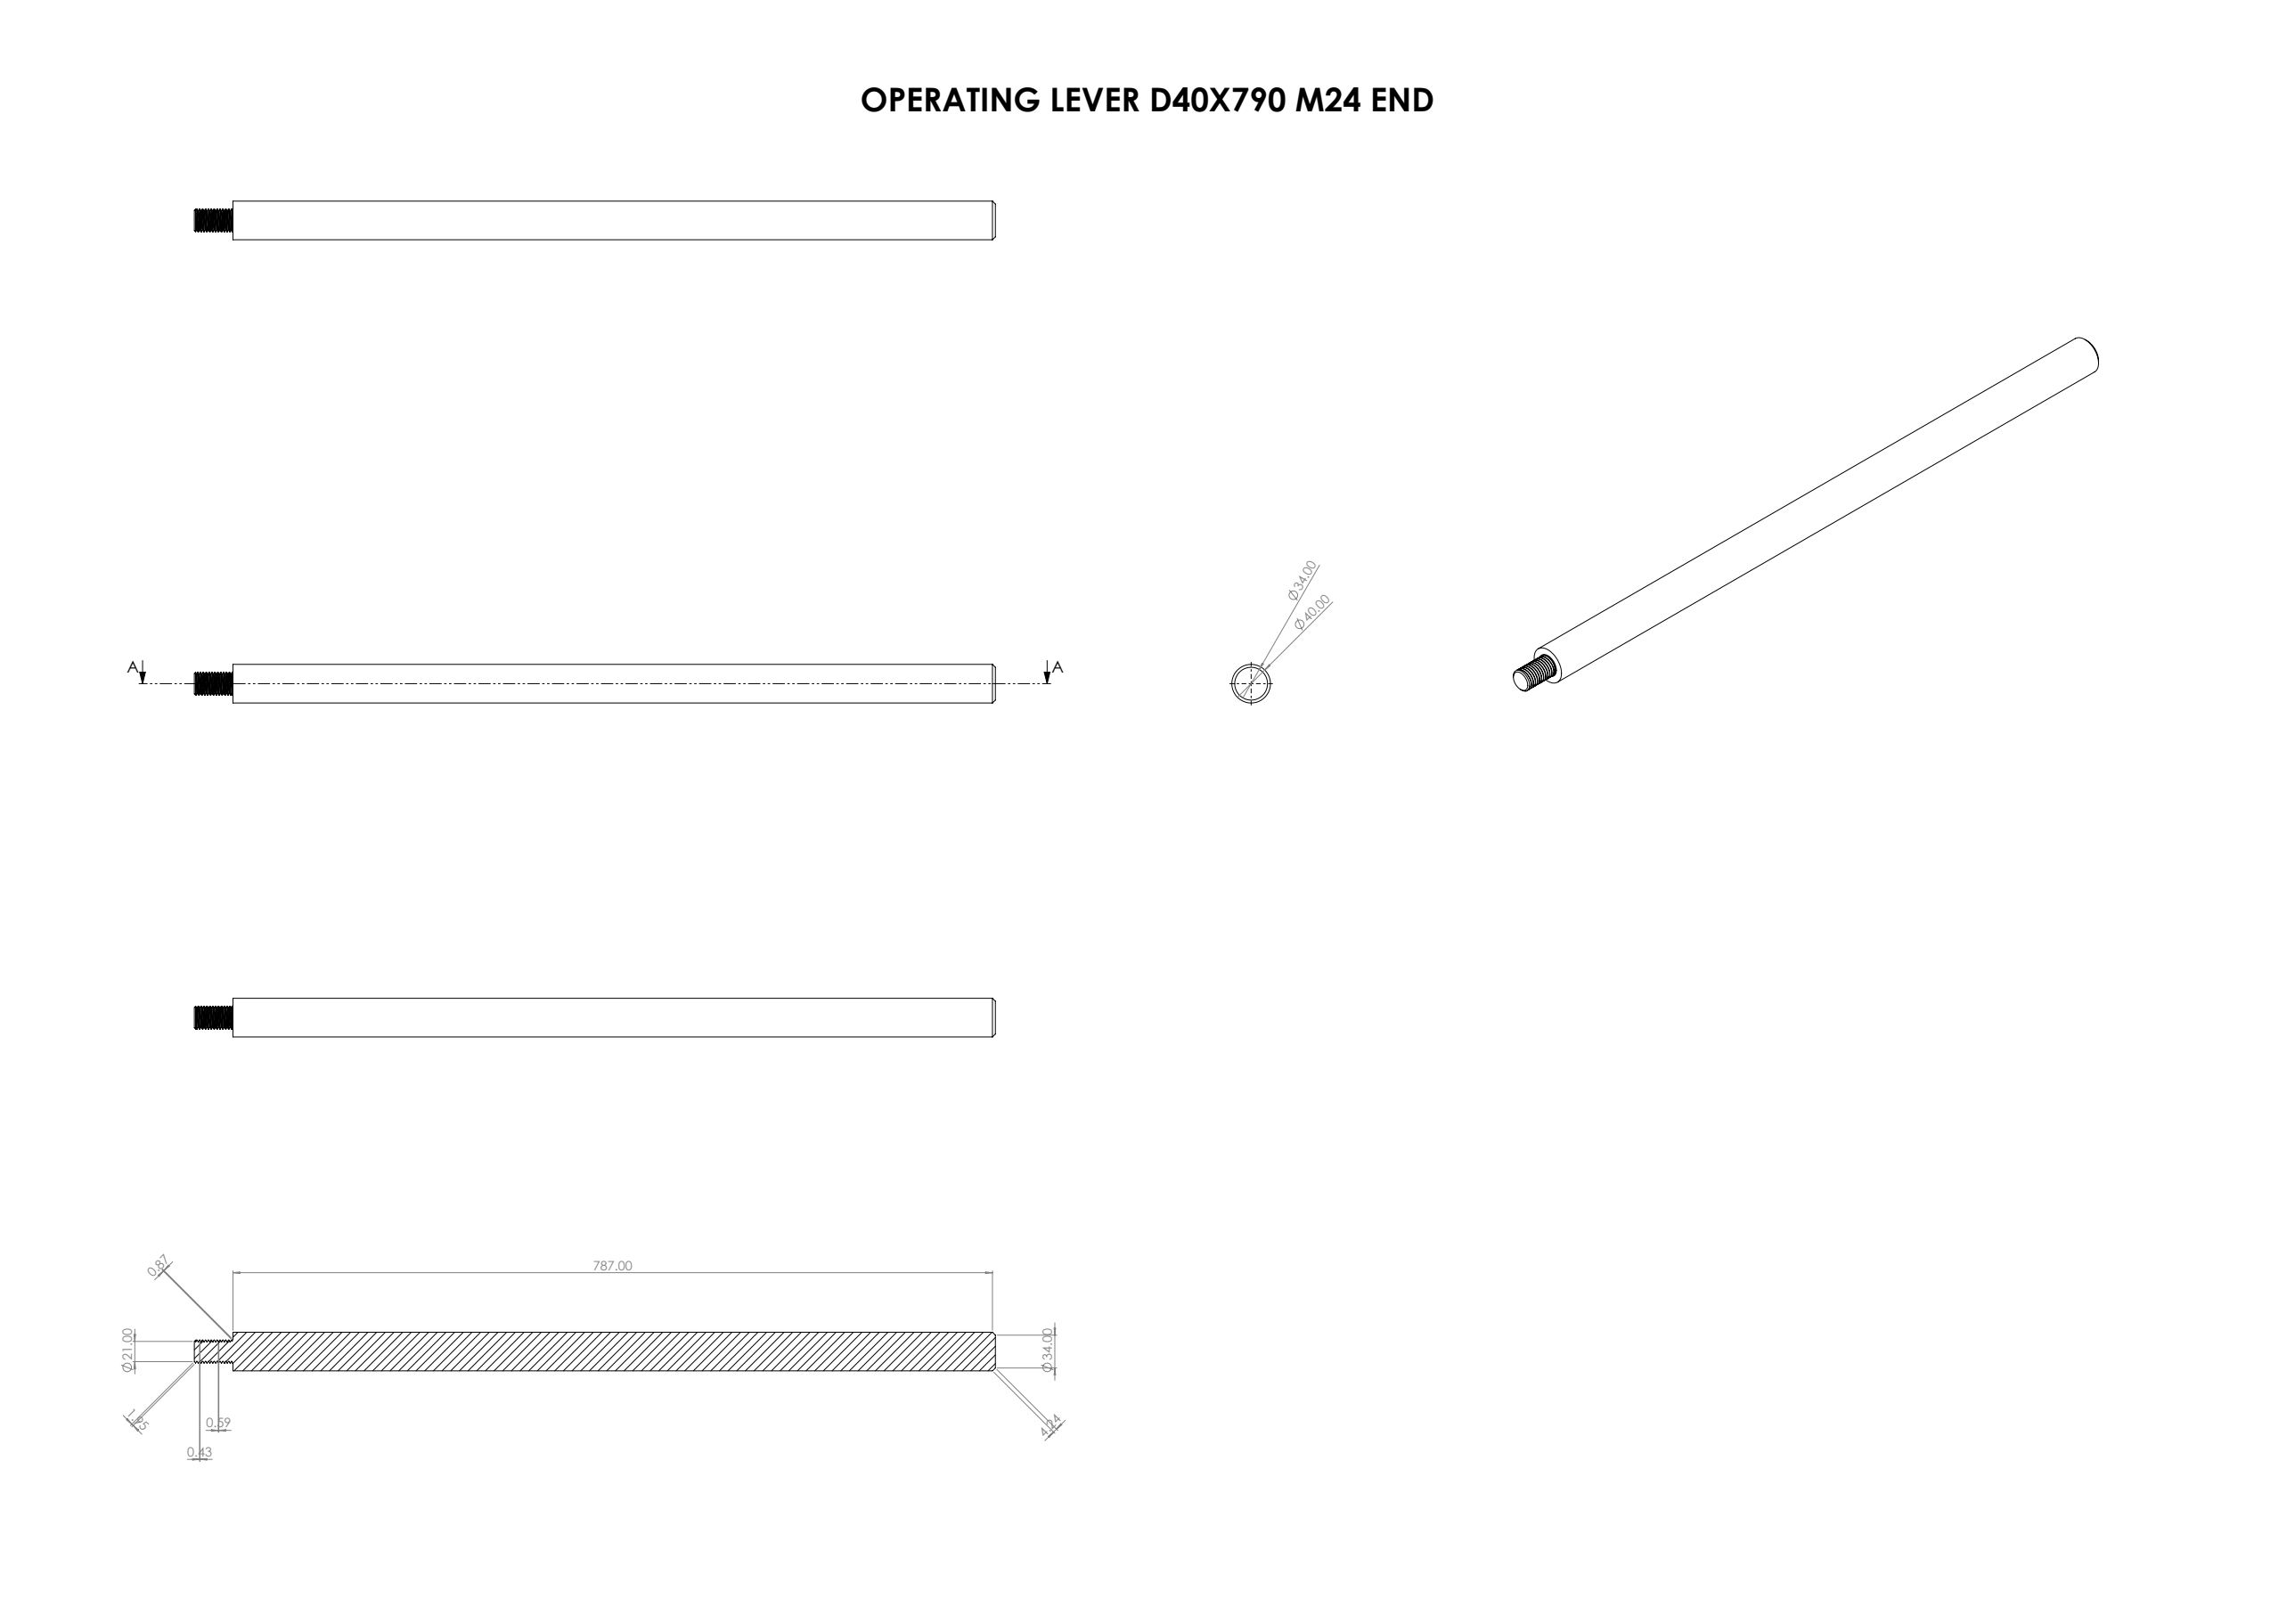
ISO-10303-21;
HEADER;
/* Generated by software containing ST-Developer
 * from STEP Tools, Inc. (www.steptools.com) 
 */

FILE_DESCRIPTION(
/* description */ (''),
/* implementation_level */ '2;1');

FILE_NAME(
/* name */ '05_Operating_Lever_D40x790_M24_End.step',
/* time_stamp */ '2026-10-19T23:58:09-07:00',
/* author */ (''),
/* organization */ (''),
/* preprocessor_version */ 'ST-DEVELOPER v20.2',
/* originating_system */ 'Autodesk Translation Framework v15.15.0.0',
/* authorisation */ '');

FILE_SCHEMA (('AP203_CONFIGURATION_CONTROLLED_3D_DESIGN_OF_MECHANICAL_PARTS_AND_ASSEMBLIES_MIM_LF { 1 0 10303 203 3 1 4 }',
'AUTOMOTIVE_DESIGN { 1 0 10303 214 3 1 1 }','INTEGRATED_CNC_SCHEMA','MODEL_BASED_INTEGRATED_MANUFACTURING_SCHEMA',
'PROCESS_PLANNING_SCHEMA','AP242_MANAGED_MODEL_BASED_3D_ENGINEERING_MIM_LF { 1 0 10303 442 3 1 4 }'));
ENDSEC;

DATA;
#10=MECHANICAL_DESIGN_GEOMETRIC_PRESENTATION_REPRESENTATION('',(#408),#70757);
#270=B_SPLINE_SURFACE_WITH_KNOTS('',3,3,((#42029,#42030,#42031,#42032,#42033,
#42034,#42035,#42036,#42037,#42038,#42039,#42040,#42041,#42042,#42043,#42044,
#42045,#42046,#42047,#42048,#42049,#42050,#42051,#42052,#42053,#42054,#42055,
#42056,#42057,#42058,#42059,#42060,#42061,#42062,#42063,#42064,#42065,#42066,
#42067,#42068,#42069,#42070,#42071,#42072,#42073,#42074,#42075,#42076,#42077,
#42078,#42079,#42080,#42081,#42082,#42083,#42084,#42085,#42086,#42087,#42088,
#42089,#42090,#42091,#42092,#42093,#42094,#42095,#42096,#42097,#42098,#42099,
#42100,#42101,#42102,#42103,#42104,#42105,#42106,#42107,#42108,#42109,#42110,
#42111,#42112,#42113,#42114,#42115,#42116,#42117,#42118,#42119,#42120,#42121,
#42122,#42123,#42124,#42125,#42126,#42127,#42128,#42129,#42130,#42131,#42132,
#42133,#42134,#42135,#42136,#42137,#42138,#42139,#42140,#42141,#42142,#42143,
#42144,#42145,#42146,#42147,#42148,#42149,#42150,#42151,#42152,#42153,#42154,
#42155,#42156,#42157,#42158,#42159,#42160,#42161,#42162,#42163,#42164,#42165,
#42166,#42167,#42168,#42169,#42170,#42171,#42172,#42173,#42174,#42175,#42176,
#42177,#42178,#42179,#42180,#42181,#42182,#42183,#42184,#42185,#42186,#42187,
#42188,#42189,#42190,#42191,#42192,#42193,#42194,#42195),(#42196,#42197,
#42198,#42199,#42200,#42201,#42202,#42203,#42204,#42205,#42206,#42207,#42208,
#42209,#42210,#42211,#42212,#42213,#42214,#42215,#42216,#42217,#42218,#42219,
#42220,#42221,#42222,#42223,#42224,#42225,#42226,#42227,#42228,#42229,#42230,
#42231,#42232,#42233,#42234,#42235,#42236,#42237,#42238,#42239,#42240,#42241,
#42242,#42243,#42244,#42245,#42246,#42247,#42248,#42249,#42250,#42251,#42252,
#42253,#42254,#42255,#42256,#42257,#42258,#42259,#42260,#42261,#42262,#42263,
#42264,#42265,#42266,#42267,#42268,#42269,#42270,#42271,#42272,#42273,#42274,
#42275,#42276,#42277,#42278,#42279,#42280,#42281,#42282,#42283,#42284,#42285,
#42286,#42287,#42288,#42289,#42290,#42291,#42292,#42293,#42294,#42295,#42296,
#42297,#42298,#42299,#42300,#42301,#42302,#42303,#42304,#42305,#42306,#42307,
#42308,#42309,#42310,#42311,#42312,#42313,#42314,#42315,#42316,#42317,#42318,
#42319,#42320,#42321,#42322,#42323,#42324,#42325,#42326,#42327,#42328,#42329,
#42330,#42331,#42332,#42333,#42334,#42335,#42336,#42337,#42338,#42339,#42340,
#42341,#42342,#42343,#42344,#42345,#42346,#42347,#42348,#42349,#42350,#42351,
#42352,#42353,#42354,#42355,#42356,#42357,#42358,#42359,#42360,#42361,#42362),
(#42363,#42364,#42365,#42366,#42367,#42368,#42369,#42370,#42371,#42372,
#42373,#42374,#42375,#42376,#42377,#42378,#42379,#42380,#42381,#42382,#42383,
#42384,#42385,#42386,#42387,#42388,#42389,#42390,#42391,#42392,#42393,#42394,
#42395,#42396,#42397,#42398,#42399,#42400,#42401,#42402,#42403,#42404,#42405,
#42406,#42407,#42408,#42409,#42410,#42411,#42412,#42413,#42414,#42415,#42416,
#42417,#42418,#42419,#42420,#42421,#42422,#42423,#42424,#42425,#42426,#42427,
#42428,#42429,#42430,#42431,#42432,#42433,#42434,#42435,#42436,#42437,#42438,
#42439,#42440,#42441,#42442,#42443,#42444,#42445,#42446,#42447,#42448,#42449,
#42450,#42451,#42452,#42453,#42454,#42455,#42456,#42457,#42458,#42459,#42460,
#42461,#42462,#42463,#42464,#42465,#42466,#42467,#42468,#42469,#42470,#42471,
#42472,#42473,#42474,#42475,#42476,#42477,#42478,#42479,#42480,#42481,#42482,
#42483,#42484,#42485,#42486,#42487,#42488,#42489,#42490,#42491,#42492,#42493,
#42494,#42495,#42496,#42497,#42498,#42499,#42500,#42501,#42502,#42503,#42504,
#42505,#42506,#42507,#42508,#42509,#42510,#42511,#42512,#42513,#42514,#42515,
#42516,#42517,#42518,#42519,#42520,#42521,#42522,#42523,#42524,#42525,#42526,
#42527,#42528,#42529),(#42530,#42531,#42532,#42533,#42534,#42535,#42536,
#42537,#42538,#42539,#42540,#42541,#42542,#42543,#42544,#42545,#42546,#42547,
#42548,#42549,#42550,#42551,#42552,#42553,#42554,#42555,#42556,#42557,#42558,
#42559,#42560,#42561,#42562,#42563,#42564,#42565,#42566,#42567,#42568,#42569,
#42570,#42571,#42572,#42573,#42574,#42575,#42576,#42577,#42578,#42579,#42580,
#42581,#42582,#42583,#42584,#42585,#42586,#42587,#42588,#42589,#42590,#42591,
#42592,#42593,#42594,#42595,#42596,#42597,#42598,#42599,#42600,#42601,#42602,
#42603,#42604,#42605,#42606,#42607,#42608,#42609,#42610,#42611,#42612,#42613,
#42614,#42615,#42616,#42617,#42618,#42619,#42620,#42621,#42622,#42623,#42624,
#42625,#42626,#42627,#42628,#42629,#42630,#42631,#42632,#42633,#42634,#42635,
#42636,#42637,#42638,#42639,#42640,#42641,#42642,#42643,#42644,#42645,#42646,
#42647,#42648,#42649,#42650,#42651,#42652,#42653,#42654,#42655,#42656,#42657,
#42658,#42659,#42660,#42661,#42662,#42663,#42664,#42665,#42666,#42667,#42668,
#42669,#42670,#42671,#42672,#42673,#42674,#42675,#42676,#42677,#42678,#42679,
#42680,#42681,#42682,#42683,#42684,#42685,#42686,#42687,#42688,#42689,#42690,
#42691,#42692,#42693,#42694,#42695,#42696)),.UNSPECIFIED.,.F.,.F.,.F.,(4,
4),(4,1,1,1,1,1,1,1,1,1,1,1,1,1,1,1,1,1,1,1,1,1,1,1,1,1,1,1,1,1,1,1,1,1,
1,1,1,1,1,1,1,1,1,1,1,1,1,1,1,1,1,1,1,1,1,1,1,1,1,1,1,1,1,1,1,1,1,1,1,1,
1,1,1,1,1,1,1,1,1,1,1,1,1,1,1,1,1,1,1,1,1,1,1,1,1,1,1,1,1,1,1,1,1,1,1,1,
1,1,1,1,1,1,1,1,1,1,1,1,1,1,1,1,1,1,1,1,1,1,1,1,1,1,1,1,1,1,1,1,1,1,1,1,
1,1,1,1,1,1,1,1,1,1,1,1,1,1,1,1,1,1,1,1,1,1,4),(0.,0.198319817466637),(8.29931545526195,
8.79726554162164,9.29521562798133,9.79316571434102,10.2911158007007,10.7890658870604,
11.2870159734201,11.7849660597798,12.2829161461395,12.7808662324992,13.2788163188589,
13.7767664052186,14.2747164915782,14.7726665779379,15.2706166642976,15.7685667506573,
16.266516837017,16.7644669233767,17.2624170097364,17.7603670960961,18.2583171824558,
18.7562672688155,19.2542173551752,19.7521674415349,20.2501175278945,20.7480676142542,
21.2460177006139,21.7439677869736,22.2419178733333,22.739867959693,23.2378180460527,
23.7357681324124,24.2337182187721,24.7316683051318,25.2296183914915,25.7275684778511,
26.2255185642108,26.7234686505705,27.2214187369302,27.7193688232899,28.2173189096496,
28.7152689960093,29.213219082369,29.7111691687287,30.2091192550884,30.7070693414481,
31.2050194278078,31.7029695141674,32.2009196005271,32.6988696868868,33.1968197732465,
33.6947698596062,34.1927199459659,34.6906700323256,35.1886201186853,35.686570205045,
36.1845202914047,36.6824703777644,37.1804204641241,37.6783705504837,38.1763206368434,
38.6742707232031,39.1722208095628,39.6701708959225,40.1681209822822,40.6660710686419,
41.1640211550016,41.6619712413613,42.159921327721,42.6578714140807,43.1558215004404,
43.6537715868,44.1517216731597,44.6496717595194,45.1476218458791,45.6455719322388,
46.1435220185985,46.6414721049582,47.1394221913179,47.6373722776776,48.1353223640373,
48.633272450397,49.1312225367567,49.6291726231163,50.127122709476,50.6250727958357,
51.1230228821954,51.6209729685551,52.1189230549148,52.6168731412745,53.1148232276342,
53.6127733139939,54.1107234003536,54.6086734867133,55.106623573073,55.6045736594326,
56.1025237457923,56.600473832152,57.0984239185117,57.5963740048714,58.0943240912311,
58.5922741775908,59.0902242639505,59.5881743503102,60.0861244366699,60.5840745230296,
61.0820246093893,61.5799746957489,62.0779247821086,62.5758748684683,63.073824954828,
63.5717750411877,64.0697251275474,64.5676752139071,65.0656253002668,65.5635753866265,
66.0615254729862,66.5594755593459,67.0574256457055,67.5553757320652,68.0533258184249,
68.5512759047846,69.0492259911443,69.547176077504,70.0451261638637,70.5430762502234,
71.0410263365831,71.5389764229428,72.0369265093025,72.5348765956622,73.0328266820218,
73.5307767683815,74.0287268547412,74.5266769411009,75.0246270274606,75.5225771138203,
76.02052720018,76.5184772865397,77.0164273728994,77.5143774592591,78.0123275456188,
78.5102776319785,79.0082277183381,79.5061778046978,80.0041278910575,80.5020779774172,
81.0000280637769,81.4979781501366,81.9959282364963,82.493878322856,82.9918284092157,
83.4897784955754,83.9877285819351,84.4856786682948,84.9836287546544,85.4815788410141,
85.9795289273738,86.4774790137335,86.9754291000932,87.4733791864529,87.9713292728126,
88.4692793591723,88.967229445532,89.4651795318917,89.9631296182514),
 .UNSPECIFIED.);
#271=B_SPLINE_SURFACE_WITH_KNOTS('',3,3,((#42914,#42915,#42916,#42917,#42918,
#42919,#42920,#42921,#42922,#42923,#42924,#42925,#42926,#42927,#42928,#42929,
#42930,#42931,#42932,#42933,#42934,#42935,#42936,#42937,#42938,#42939,#42940,
#42941,#42942,#42943,#42944,#42945,#42946,#42947,#42948,#42949,#42950,#42951,
#42952,#42953,#42954,#42955,#42956,#42957,#42958,#42959,#42960,#42961,#42962,
#42963,#42964,#42965,#42966,#42967,#42968,#42969,#42970,#42971,#42972,#42973,
#42974,#42975,#42976,#42977,#42978,#42979,#42980,#42981,#42982,#42983,#42984,
#42985,#42986,#42987,#42988,#42989,#42990,#42991,#42992,#42993,#42994,#42995,
#42996,#42997,#42998,#42999,#43000,#43001,#43002,#43003,#43004,#43005,#43006,
#43007,#43008,#43009,#43010,#43011,#43012,#43013,#43014,#43015,#43016,#43017,
#43018,#43019,#43020,#43021,#43022,#43023,#43024,#43025,#43026,#43027,#43028,
#43029,#43030,#43031,#43032,#43033,#43034,#43035,#43036,#43037,#43038,#43039,
#43040,#43041,#43042,#43043,#43044,#43045,#43046,#43047,#43048,#43049,#43050,
#43051,#43052,#43053,#43054,#43055,#43056,#43057,#43058,#43059,#43060,#43061,
#43062,#43063,#43064,#43065,#43066,#43067,#43068,#43069,#43070,#43071,#43072,
#43073,#43074,#43075,#43076,#43077,#43078,#43079,#43080),(#43081,#43082,
#43083,#43084,#43085,#43086,#43087,#43088,#43089,#43090,#43091,#43092,#43093,
#43094,#43095,#43096,#43097,#43098,#43099,#43100,#43101,#43102,#43103,#43104,
#43105,#43106,#43107,#43108,#43109,#43110,#43111,#43112,#43113,#43114,#43115,
#43116,#43117,#43118,#43119,#43120,#43121,#43122,#43123,#43124,#43125,#43126,
#43127,#43128,#43129,#43130,#43131,#43132,#43133,#43134,#43135,#43136,#43137,
#43138,#43139,#43140,#43141,#43142,#43143,#43144,#43145,#43146,#43147,#43148,
#43149,#43150,#43151,#43152,#43153,#43154,#43155,#43156,#43157,#43158,#43159,
#43160,#43161,#43162,#43163,#43164,#43165,#43166,#43167,#43168,#43169,#43170,
#43171,#43172,#43173,#43174,#43175,#43176,#43177,#43178,#43179,#43180,#43181,
#43182,#43183,#43184,#43185,#43186,#43187,#43188,#43189,#43190,#43191,#43192,
#43193,#43194,#43195,#43196,#43197,#43198,#43199,#43200,#43201,#43202,#43203,
#43204,#43205,#43206,#43207,#43208,#43209,#43210,#43211,#43212,#43213,#43214,
#43215,#43216,#43217,#43218,#43219,#43220,#43221,#43222,#43223,#43224,#43225,
#43226,#43227,#43228,#43229,#43230,#43231,#43232,#43233,#43234,#43235,#43236,
#43237,#43238,#43239,#43240,#43241,#43242,#43243,#43244,#43245,#43246,#43247),
(#43248,#43249,#43250,#43251,#43252,#43253,#43254,#43255,#43256,#43257,
#43258,#43259,#43260,#43261,#43262,#43263,#43264,#43265,#43266,#43267,#43268,
#43269,#43270,#43271,#43272,#43273,#43274,#43275,#43276,#43277,#43278,#43279,
#43280,#43281,#43282,#43283,#43284,#43285,#43286,#43287,#43288,#43289,#43290,
#43291,#43292,#43293,#43294,#43295,#43296,#43297,#43298,#43299,#43300,#43301,
#43302,#43303,#43304,#43305,#43306,#43307,#43308,#43309,#43310,#43311,#43312,
#43313,#43314,#43315,#43316,#43317,#43318,#43319,#43320,#43321,#43322,#43323,
#43324,#43325,#43326,#43327,#43328,#43329,#43330,#43331,#43332,#43333,#43334,
#43335,#43336,#43337,#43338,#43339,#43340,#43341,#43342,#43343,#43344,#43345,
#43346,#43347,#43348,#43349,#43350,#43351,#43352,#43353,#43354,#43355,#43356,
#43357,#43358,#43359,#43360,#43361,#43362,#43363,#43364,#43365,#43366,#43367,
#43368,#43369,#43370,#43371,#43372,#43373,#43374,#43375,#43376,#43377,#43378,
#43379,#43380,#43381,#43382,#43383,#43384,#43385,#43386,#43387,#43388,#43389,
#43390,#43391,#43392,#43393,#43394,#43395,#43396,#43397,#43398,#43399,#43400,
#43401,#43402,#43403,#43404,#43405,#43406,#43407,#43408,#43409,#43410,#43411,
#43412,#43413,#43414),(#43415,#43416,#43417,#43418,#43419,#43420,#43421,
#43422,#43423,#43424,#43425,#43426,#43427,#43428,#43429,#43430,#43431,#43432,
#43433,#43434,#43435,#43436,#43437,#43438,#43439,#43440,#43441,#43442,#43443,
#43444,#43445,#43446,#43447,#43448,#43449,#43450,#43451,#43452,#43453,#43454,
#43455,#43456,#43457,#43458,#43459,#43460,#43461,#43462,#43463,#43464,#43465,
#43466,#43467,#43468,#43469,#43470,#43471,#43472,#43473,#43474,#43475,#43476,
#43477,#43478,#43479,#43480,#43481,#43482,#43483,#43484,#43485,#43486,#43487,
#43488,#43489,#43490,#43491,#43492,#43493,#43494,#43495,#43496,#43497,#43498,
#43499,#43500,#43501,#43502,#43503,#43504,#43505,#43506,#43507,#43508,#43509,
#43510,#43511,#43512,#43513,#43514,#43515,#43516,#43517,#43518,#43519,#43520,
#43521,#43522,#43523,#43524,#43525,#43526,#43527,#43528,#43529,#43530,#43531,
#43532,#43533,#43534,#43535,#43536,#43537,#43538,#43539,#43540,#43541,#43542,
#43543,#43544,#43545,#43546,#43547,#43548,#43549,#43550,#43551,#43552,#43553,
#43554,#43555,#43556,#43557,#43558,#43559,#43560,#43561,#43562,#43563,#43564,
#43565,#43566,#43567,#43568,#43569,#43570,#43571,#43572,#43573,#43574,#43575,
#43576,#43577,#43578,#43579,#43580,#43581)),.UNSPECIFIED.,.F.,.F.,.F.,(4,
4),(4,1,1,1,1,1,1,1,1,1,1,1,1,1,1,1,1,1,1,1,1,1,1,1,1,1,1,1,1,1,1,1,1,1,
1,1,1,1,1,1,1,1,1,1,1,1,1,1,1,1,1,1,1,1,1,1,1,1,1,1,1,1,1,1,1,1,1,1,1,1,
1,1,1,1,1,1,1,1,1,1,1,1,1,1,1,1,1,1,1,1,1,1,1,1,1,1,1,1,1,1,1,1,1,1,1,1,
1,1,1,1,1,1,1,1,1,1,1,1,1,1,1,1,1,1,1,1,1,1,1,1,1,1,1,1,1,1,1,1,1,1,1,1,
1,1,1,1,1,1,1,1,1,1,1,1,1,1,1,1,1,1,1,1,1,1,4),(0.,0.198319817466637),(11.6150328478181,
12.1129829341778,12.6109330205375,13.1088831068972,13.6068331932569,14.1047832796166,
14.6027333659763,15.100683452336,15.5986335386957,16.0965836250554,16.594533711415,
17.0924837977747,17.5904338841344,18.0883839704941,18.5863340568538,19.0842841432135,
19.5822342295732,20.0801843159329,20.5781344022926,21.0760844886523,21.574034575012,
22.0719846613717,22.5699347477313,23.067884834091,23.5658349204507,24.0637850068104,
24.5617350931701,25.0596851795298,25.5576352658895,26.0555853522492,26.5535354386089,
27.0514855249686,27.5494356113283,28.047385697688,28.5453357840476,29.0432858704073,
29.541235956767,30.0391860431267,30.5371361294864,31.0350862158461,31.5330363022058,
32.0309863885655,32.5289364749252,33.0268865612849,33.5248366476446,34.0227867340043,
34.520736820364,35.0186869067236,35.5166369930833,36.014587079443,36.5125371658027,
37.0104872521624,37.5084373385221,38.0063874248818,38.5043375112415,39.0022875976012,
39.5002376839609,39.9981877703206,40.4961378566802,40.9940879430399,41.4920380293996,
41.9899881157593,42.487938202119,42.9858882884787,43.4838383748384,43.9817884611981,
44.4797385475578,44.9776886339175,45.4756387202772,45.9735888066369,46.4715388929966,
46.9694889793562,47.4674390657159,47.9653891520756,48.4633392384353,48.961289324795,
49.4592394111547,49.9571894975144,50.4551395838741,50.9530896702338,51.4510397565935,
51.9489898429532,52.4469399293129,52.9448900156726,53.4428401020322,53.9407901883919,
54.4387402747516,54.9366903611113,55.434640447471,55.9325905338307,56.4305406201904,
56.9284907065501,57.4264407929098,57.9243908792695,58.4223409656292,58.9202910519889,
59.4182411383485,59.9161912247082,60.4141413110679,60.9120913974276,61.4100414837873,
61.907991570147,62.4059416565067,62.9038917428664,63.4018418292261,63.8997919155858,
64.3977420019455,64.8956920883052,65.3936421746648,65.8915922610245,66.3895423473842,
66.8874924337439,67.3854425201036,67.8833926064633,68.381342692823,68.8792927791827,
69.3772428655424,69.8751929519021,70.3731430382618,70.8710931246215,71.3690432109811,
71.8669932973408,72.3649433837005,72.8628934700602,73.3608435564199,73.8587936427796,
74.3567437291393,74.854693815499,75.3526439018587,75.8505939882184,76.3485440745781,
76.8464941609378,77.3444442472975,77.8423943336572,78.3403444200168,78.8382945063765,
79.3362445927362,79.8341946790959,80.3321447654556,80.8300948518153,81.328044938175,
81.8259950245347,82.3239451108944,82.8218951972541,83.3198452836138,83.8177953699735,
84.3157454563331,84.8136955426928,85.3116456290525,85.8095957154122,86.3075458017719,
86.8054958881316,87.3034459744913,87.801396060851,88.2993461472107,88.7972962335704,
89.2952463199301,89.7931964062898,90.2911464926494,90.7890965790091,91.2870466653688,
91.7849967517285,92.2829468380882,92.7808969244479,93.2788470108076),
 .UNSPECIFIED.);
#378=SHAPE_REPRESENTATION_RELATIONSHIP('SRR','None',#70819,#393);
#393=ADVANCED_BREP_SHAPE_REPRESENTATION('',(#468),#70743);
#408=STYLED_ITEM('',(#71061),#468);
#468=MANIFOLD_SOLID_BREP('Lever',#26873);
#558=CYLINDRICAL_SURFACE('',#27232,1.188225);
#559=CYLINDRICAL_SURFACE('',#27234,1.188225);
#560=CYLINDRICAL_SURFACE('',#27235,1.188225);
#561=CYLINDRICAL_SURFACE('',#27236,1.188225);
#562=CYLINDRICAL_SURFACE('',#27237,1.188225);
#563=CYLINDRICAL_SURFACE('',#27238,1.188225);
#564=CYLINDRICAL_SURFACE('',#27239,1.188225);
#565=CYLINDRICAL_SURFACE('',#27240,1.188225);
#566=CYLINDRICAL_SURFACE('',#27241,1.188225);
#567=CYLINDRICAL_SURFACE('',#27242,1.188225);
#568=CYLINDRICAL_SURFACE('',#27243,1.188225);
#569=CYLINDRICAL_SURFACE('',#27244,1.188225);
#570=CYLINDRICAL_SURFACE('',#27245,1.188225);
#571=CYLINDRICAL_SURFACE('',#27246,1.016475);
#572=CYLINDRICAL_SURFACE('',#27248,1.016475);
#573=CYLINDRICAL_SURFACE('',#27250,1.016475);
#574=CYLINDRICAL_SURFACE('',#27251,1.016475);
#575=CYLINDRICAL_SURFACE('',#27252,1.016475);
#576=CYLINDRICAL_SURFACE('',#27253,1.016475);
#577=CYLINDRICAL_SURFACE('',#27254,1.016475);
#578=CYLINDRICAL_SURFACE('',#27255,1.016475);
#579=CYLINDRICAL_SURFACE('',#27256,1.016475);
#580=CYLINDRICAL_SURFACE('',#27257,1.016475);
#581=CYLINDRICAL_SURFACE('',#27258,1.016475);
#582=CYLINDRICAL_SURFACE('',#27259,1.016475);
#583=CYLINDRICAL_SURFACE('',#27260,1.016475);
#584=CYLINDRICAL_SURFACE('',#27268,1.016475);
#585=CYLINDRICAL_SURFACE('',#27269,1.188225);
#586=CYLINDRICAL_SURFACE('',#27275,2.);
#849=FACE_BOUND('',#4223,.T.);
#1035=B_SPLINE_CURVE_WITH_KNOTS('',3,(#40328,#40329,#40330,#40331,#40332,
#40333,#40334,#40335,#40336,#40337,#40338,#40339,#40340,#40341,#40342,#40343),
 .UNSPECIFIED.,.F.,.F.,(4,3,3,3,3,4),(-4.09293042013078,-3.98360069087754,
-3.48565060451784,-2.98770051815815,-2.48975043179846,-2.07680027204821),
 .UNSPECIFIED.);
#1036=B_SPLINE_CURVE_WITH_KNOTS('',3,(#40346,#40347,#40348,#40349,#40350,
#40351,#40352,#40353,#40354,#40355),.UNSPECIFIED.,.F.,.F.,(4,3,3,4),(0.,
0.497950086359684,0.995900172719378,1.12546250550734),.UNSPECIFIED.);
#1037=B_SPLINE_CURVE_WITH_KNOTS('',3,(#40360,#40361,#40362,#40363,#40364,
#40365,#40366,#40367,#40368,#40369,#40370,#40371,#40372,#40373,#40374,#40375,
#40376,#40377,#40378,#40379,#40380,#40381,#40382,#40383,#40384,#40385,#40386,
#40387,#40388,#40389,#40390,#40391,#40392,#40393,#40394,#40395,#40396,#40397,
#40398,#40399),.UNSPECIFIED.,.F.,.F.,(4,3,3,3,3,3,3,3,3,3,3,3,3,4),(-10.3761157273103,
-9.95900172719384,-9.46105164083415,-8.96310155447445,-8.46515146811476,
-7.96720138175507,-7.46925129539538,-6.97130120903569,-6.473351122676,-5.9754010363163,
-5.47745094995661,-4.97950086359692,-4.48155077723723,-4.09293042013078),
 .UNSPECIFIED.);
#1038=B_SPLINE_CURVE_WITH_KNOTS('',3,(#40400,#40401,#40402,#40403,#40404,
#40405,#40406,#40407,#40408,#40409,#40410,#40411,#40412,#40413,#40414,#40415,
#40416,#40417,#40418,#40419,#40420,#40421,#40422,#40423,#40424,#40425,#40426,
#40427,#40428,#40429,#40430,#40431,#40432,#40433,#40434,#40435,#40436,#40437,
#40438,#40439),.UNSPECIFIED.,.F.,.F.,(4,3,3,3,3,3,3,3,3,3,3,3,3,4),(1.12546250550734,
1.49385025907907,1.99180034543876,2.48975043179845,2.98770051815815,3.48565060451784,
3.98360069087753,4.48155077723722,4.97950086359691,5.47745094995661,5.9754010363163,
6.47335112267599,6.97130120903568,7.40864781268687),.UNSPECIFIED.);
#1039=B_SPLINE_CURVE_WITH_KNOTS('',3,(#40444,#40445,#40446,#40447,#40448,
#40449,#40450,#40451,#40452,#40453,#40454,#40455,#40456,#40457,#40458,#40459,
#40460,#40461,#40462,#40463,#40464,#40465,#40466,#40467,#40468,#40469,#40470,
#40471,#40472,#40473,#40474,#40475,#40476,#40477,#40478,#40479,#40480,#40481,
#40482,#40483,#40484,#40485,#40486),.UNSPECIFIED.,.F.,.F.,(4,3,3,3,3,3,
3,3,3,3,3,3,3,3,4),(-16.65930103449,-16.4323528498698,-15.9344027635101,
-15.4364526771504,-14.9385025907908,-14.4405525044311,-13.9426024180714,
-13.4446523317117,-12.946702245352,-12.4487521589923,-11.9508020726326,
-11.4528519862729,-10.9549018999132,-10.4569518135535,-10.3761157273103),
 .UNSPECIFIED.);
#1040=B_SPLINE_CURVE_WITH_KNOTS('',3,(#40487,#40488,#40489,#40490,#40491,
#40492,#40493,#40494,#40495,#40496,#40497,#40498,#40499,#40500,#40501,#40502,
#40503,#40504,#40505,#40506,#40507,#40508,#40509,#40510,#40511,#40512,#40513,
#40514,#40515,#40516,#40517,#40518,#40519,#40520,#40521,#40522,#40523,#40524,
#40525,#40526,#40527,#40528,#40529),.UNSPECIFIED.,.F.,.F.,(4,3,3,3,3,3,
3,3,3,3,3,3,3,3,4),(7.40864781268687,7.46925129539537,7.96720138175506,
8.46515146811476,8.96310155447445,9.46105164083414,9.95900172719383,10.4569518135535,
10.9549018999132,11.4528519862729,11.9508020726326,12.4487521589923,12.946702245352,
13.4446523317117,13.6918331198665),.UNSPECIFIED.);
#1041=B_SPLINE_CURVE_WITH_KNOTS('',3,(#40534,#40535,#40536,#40537,#40538,
#40539,#40540,#40541,#40542,#40543,#40544,#40545,#40546,#40547,#40548,#40549,
#40550,#40551,#40552,#40553,#40554,#40555,#40556,#40557,#40558,#40559,#40560,
#40561,#40562,#40563,#40564,#40565,#40566,#40567,#40568,#40569,#40570,#40571,
#40572,#40573,#40574,#40575,#40576),.UNSPECIFIED.,.F.,.F.,(4,3,3,3,3,3,
3,3,3,3,3,3,3,3,4),(-22.9424863416695,-22.9057039725458,-22.4077538861861,
-21.9098037998264,-21.4118537134668,-20.9139036271071,-20.4159535407474,
-19.9180034543877,-19.420053368028,-18.9221032816683,-18.4241531953086,
-17.9262031089489,-17.4282530225892,-16.9303029362295,-16.65930103449),
 .UNSPECIFIED.);
#1042=B_SPLINE_CURVE_WITH_KNOTS('',3,(#40577,#40578,#40579,#40580,#40581,
#40582,#40583,#40584,#40585,#40586,#40587,#40588,#40589,#40590,#40591,#40592,
#40593,#40594,#40595,#40596,#40597,#40598,#40599,#40600,#40601,#40602,#40603,
#40604,#40605,#40606,#40607,#40608,#40609,#40610,#40611,#40612,#40613,#40614,
#40615,#40616,#40617,#40618,#40619),.UNSPECIFIED.,.F.,.F.,(4,3,3,3,3,3,
3,3,3,3,3,3,3,3,4),(13.6918331198665,13.9426024180714,14.4405525044311,
14.9385025907907,15.4364526771504,15.9344027635101,16.4323528498698,16.9303029362295,
17.4282530225892,17.9262031089489,18.4241531953086,18.9221032816683,19.420053368028,
19.9180034543877,19.9750184270461),.UNSPECIFIED.);
#1043=B_SPLINE_CURVE_WITH_KNOTS('',3,(#40624,#40625,#40626,#40627,#40628,
#40629,#40630,#40631,#40632,#40633,#40634,#40635,#40636,#40637,#40638,#40639,
#40640,#40641,#40642,#40643,#40644,#40645,#40646,#40647,#40648,#40649,#40650,
#40651,#40652,#40653,#40654,#40655,#40656,#40657,#40658,#40659,#40660,#40661,
#40662,#40663),.UNSPECIFIED.,.F.,.F.,(4,3,3,3,3,3,3,3,3,3,3,3,3,4),(-29.2256716488492,
-28.8811050088621,-28.3831549225024,-27.8852048361428,-27.3872547497831,
-26.8893046634234,-26.3913545770637,-25.893404490704,-25.3954544043443,
-24.8975043179846,-24.3995542316249,-23.9016041452652,-23.4036540589055,
-22.9424863416695),.UNSPECIFIED.);
#1044=B_SPLINE_CURVE_WITH_KNOTS('',3,(#40664,#40665,#40666,#40667,#40668,
#40669,#40670,#40671,#40672,#40673,#40674,#40675,#40676,#40677,#40678,#40679,
#40680,#40681,#40682,#40683,#40684,#40685,#40686,#40687,#40688,#40689,#40690,
#40691,#40692,#40693,#40694,#40695,#40696,#40697,#40698,#40699,#40700,#40701,
#40702,#40703),.UNSPECIFIED.,.F.,.F.,(4,3,3,3,3,3,3,3,3,3,3,3,3,4),(19.9750184270461,
20.4159535407473,20.913903627107,21.4118537134667,21.9098037998264,22.4077538861861,
22.9057039725458,23.4036540589055,23.9016041452652,24.3995542316249,24.8975043179846,
25.3954544043443,25.893404490704,26.2582037342256),.UNSPECIFIED.);
#1045=B_SPLINE_CURVE_WITH_KNOTS('',3,(#40708,#40709,#40710,#40711,#40712,
#40713,#40714,#40715,#40716,#40717,#40718,#40719,#40720,#40721,#40722,#40723,
#40724,#40725,#40726,#40727,#40728,#40729,#40730,#40731,#40732,#40733,#40734,
#40735,#40736,#40737,#40738,#40739,#40740,#40741,#40742,#40743,#40744,#40745,
#40746,#40747,#40748,#40749,#40750),.UNSPECIFIED.,.F.,.F.,(4,3,3,3,3,3,
3,3,3,3,3,3,3,3,4),(-35.5088569560287,-35.3544561315381,-34.8565060451784,
-34.3585559588187,-33.860605872459,-33.3626557860994,-32.8647056997397,
-32.36675561338,-31.8688055270203,-31.3708554406606,-30.8729053543009,-30.3749552679412,
-29.8770051815815,-29.3790550952218,-29.2256716488492),.UNSPECIFIED.);
#1046=B_SPLINE_CURVE_WITH_KNOTS('',3,(#40751,#40752,#40753,#40754,#40755,
#40756,#40757,#40758,#40759,#40760,#40761,#40762,#40763,#40764,#40765,#40766,
#40767,#40768,#40769,#40770,#40771,#40772,#40773,#40774,#40775,#40776,#40777,
#40778,#40779,#40780,#40781,#40782,#40783,#40784,#40785,#40786,#40787,#40788,
#40789,#40790,#40791,#40792,#40793),.UNSPECIFIED.,.F.,.F.,(4,3,3,3,3,3,
3,3,3,3,3,3,3,3,4),(26.2582037342256,26.3913545770637,26.8893046634233,
27.387254749783,27.8852048361427,28.3831549225024,28.8811050088621,29.3790550952218,
29.8770051815815,30.3749552679412,30.8729053543009,31.3708554406606,31.8688055270203,
32.3667556133799,32.5413890414053),.UNSPECIFIED.);
#1047=B_SPLINE_CURVE_WITH_KNOTS('',3,(#40798,#40799,#40800,#40801,#40802,
#40803,#40804,#40805,#40806,#40807,#40808,#40809,#40810,#40811,#40812,#40813,
#40814,#40815,#40816,#40817,#40818,#40819,#40820,#40821,#40822,#40823,#40824,
#40825,#40826,#40827,#40828,#40829,#40830,#40831,#40832,#40833,#40834,#40835,
#40836,#40837),.UNSPECIFIED.,.F.,.F.,(4,3,3,3,3,3,3,3,3,3,3,3,3,4),(-41.7920422632082,
-41.3298571678544,-40.8319070814947,-40.333956995135,-39.8360069087754,
-39.3380568224157,-38.840106736056,-38.3421566496963,-37.8442065633366,
-37.3462564769769,-36.8483063906172,-36.3503563042575,-35.8524062178978,
-35.5088569560287),.UNSPECIFIED.);
#1048=B_SPLINE_CURVE_WITH_KNOTS('',3,(#40838,#40839,#40840,#40841,#40842,
#40843,#40844,#40845,#40846,#40847,#40848,#40849,#40850,#40851,#40852,#40853,
#40854,#40855,#40856,#40857,#40858,#40859,#40860,#40861,#40862,#40863,#40864,
#40865,#40866,#40867,#40868,#40869,#40870,#40871,#40872,#40873,#40874,#40875,
#40876,#40877),.UNSPECIFIED.,.F.,.F.,(4,3,3,3,3,3,3,3,3,3,3,3,3,4),(32.5413890414053,
32.8647056997396,33.3626557860993,33.860605872459,34.3585559588187,34.8565060451784,
35.3544561315381,35.8524062178978,36.3503563042575,36.8483063906172,37.3462564769769,
37.8442065633366,38.3421566496963,38.8245743485848),.UNSPECIFIED.);
#1049=B_SPLINE_CURVE_WITH_KNOTS('',3,(#40882,#40883,#40884,#40885,#40886,
#40887,#40888,#40889,#40890,#40891,#40892,#40893,#40894,#40895,#40896,#40897,
#40898,#40899,#40900,#40901,#40902,#40903,#40904,#40905,#40906,#40907,#40908,
#40909,#40910,#40911,#40912,#40913,#40914,#40915,#40916,#40917,#40918,#40919,
#40920,#40921,#40922,#40923,#40924),.UNSPECIFIED.,.F.,.F.,(4,3,3,3,3,3,
3,3,3,3,3,3,3,3,4),(-48.0752275703879,-47.8032082905304,-47.3052582041707,
-46.807308117811,-46.3093580314513,-45.8114079450917,-45.313457858732,-44.8155077723723,
-44.3175576860126,-43.8196075996529,-43.3216575132932,-42.8237074269335,
-42.3257573405738,-41.8278072542141,-41.7920422632082),.UNSPECIFIED.);
#1050=B_SPLINE_CURVE_WITH_KNOTS('',3,(#40925,#40926,#40927,#40928,#40929,
#40930,#40931,#40932,#40933,#40934,#40935,#40936,#40937,#40938,#40939,#40940,
#40941,#40942,#40943,#40944,#40945,#40946,#40947,#40948,#40949,#40950,#40951,
#40952,#40953,#40954,#40955,#40956,#40957,#40958,#40959,#40960,#40961,#40962,
#40963,#40964,#40965,#40966,#40967),.UNSPECIFIED.,.F.,.F.,(4,3,3,3,3,3,
3,3,3,3,3,3,3,3,4),(38.8245743485848,38.8401067360559,39.3380568224156,
39.8360069087753,40.333956995135,40.8319070814947,41.3298571678544,41.8278072542141,
42.3257573405738,42.8237074269335,43.3216575132932,43.8196075996529,44.3175576860125,
44.8155077723722,45.1077596557645),.UNSPECIFIED.);
#1051=B_SPLINE_CURVE_WITH_KNOTS('',3,(#40972,#40973,#40974,#40975,#40976,
#40977,#40978,#40979,#40980,#40981,#40982,#40983,#40984,#40985,#40986,#40987,
#40988,#40989,#40990,#40991,#40992,#40993,#40994,#40995,#40996,#40997,#40998,
#40999,#41000,#41001,#41002,#41003,#41004,#41005,#41006,#41007,#41008,#41009,
#41010,#41011,#41012,#41013,#41014),.UNSPECIFIED.,.F.,.F.,(4,3,3,3,3,3,
3,3,3,3,3,3,3,3,4),(-54.3584128775674,-54.2765594132064,-53.7786093268467,
-53.280659240487,-52.7827091541273,-52.2847590677677,-51.786808981408,-51.2888588950483,
-50.7909088086886,-50.2929587223289,-49.7950086359692,-49.2970585496095,
-48.7991084632498,-48.3011583768901,-48.0752275703879),.UNSPECIFIED.);
#1052=B_SPLINE_CURVE_WITH_KNOTS('',3,(#41015,#41016,#41017,#41018,#41019,
#41020,#41021,#41022,#41023,#41024,#41025,#41026,#41027,#41028,#41029,#41030,
#41031,#41032,#41033,#41034,#41035,#41036,#41037,#41038,#41039,#41040,#41041,
#41042,#41043,#41044,#41045,#41046,#41047,#41048,#41049,#41050,#41051,#41052,
#41053,#41054,#41055,#41056,#41057),.UNSPECIFIED.,.F.,.F.,(4,3,3,3,3,3,
3,3,3,3,3,3,3,3,4),(45.1077596557645,45.3134578587319,45.8114079450916,
46.3093580314513,46.807308117811,47.3052582041707,47.8032082905304,48.3011583768901,
48.7991084632498,49.2970585496095,49.7950086359692,50.2929587223289,50.7909088086885,
51.2888588950482,51.390944962944),.UNSPECIFIED.);
#1053=B_SPLINE_CURVE_WITH_KNOTS('',3,(#41062,#41063,#41064,#41065,#41066,
#41067,#41068,#41069,#41070,#41071,#41072,#41073,#41074,#41075,#41076,#41077,
#41078,#41079,#41080,#41081,#41082,#41083,#41084,#41085,#41086,#41087,#41088,
#41089,#41090,#41091,#41092,#41093,#41094,#41095,#41096,#41097,#41098,#41099,
#41100,#41101),.UNSPECIFIED.,.F.,.F.,(4,3,3,3,3,3,3,3,3,3,3,3,3,4),(-60.6415981847471,
-60.2519604495227,-59.754010363163,-59.2560602768033,-58.7581101904437,
-58.260160104084,-57.7622100177243,-57.2642599313646,-56.7663098450049,
-56.2683597586452,-55.7704096722855,-55.2724595859258,-54.7745094995661,
-54.3584128775674),.UNSPECIFIED.);
#1054=B_SPLINE_CURVE_WITH_KNOTS('',3,(#41102,#41103,#41104,#41105,#41106,
#41107,#41108,#41109,#41110,#41111,#41112,#41113,#41114,#41115,#41116,#41117,
#41118,#41119,#41120,#41121,#41122,#41123,#41124,#41125,#41126,#41127,#41128,
#41129,#41130,#41131,#41132,#41133,#41134,#41135,#41136,#41137,#41138,#41139,
#41140,#41141),.UNSPECIFIED.,.F.,.F.,(4,3,3,3,3,3,3,3,3,3,3,3,3,4),(51.390944962944,
51.7868089814079,52.2847590677676,52.7827091541273,53.280659240487,53.7786093268467,
54.2765594132064,54.7745094995661,55.2724595859258,55.7704096722855,56.2683597586451,
56.7663098450048,57.2642599313645,57.6741302701237),.UNSPECIFIED.);
#1055=B_SPLINE_CURVE_WITH_KNOTS('',3,(#41146,#41147,#41148,#41149,#41150,
#41151,#41152,#41153,#41154,#41155,#41156,#41157,#41158,#41159,#41160,#41161,
#41162,#41163,#41164,#41165,#41166,#41167,#41168,#41169,#41170,#41171,#41172,
#41173,#41174,#41175,#41176,#41177,#41178,#41179,#41180,#41181,#41182,#41183,
#41184,#41185,#41186,#41187,#41188),.UNSPECIFIED.,.F.,.F.,(4,3,3,3,3,3,
3,3,3,3,3,3,3,3,4),(-66.9247834919266,-66.7253115721987,-66.227361485839,
-65.7294113994793,-65.2314613131196,-64.73351122676,-64.2355611404003,-63.7376110540406,
-63.2396609676809,-62.7417108813212,-62.2437607949615,-61.7458107086018,
-61.2478606222421,-60.7499105358824,-60.6415981847471),.UNSPECIFIED.);
#1056=B_SPLINE_CURVE_WITH_KNOTS('',3,(#41189,#41190,#41191,#41192,#41193,
#41194,#41195,#41196,#41197,#41198,#41199,#41200,#41201,#41202,#41203,#41204,
#41205,#41206,#41207,#41208,#41209,#41210,#41211,#41212,#41213,#41214,#41215,
#41216,#41217,#41218,#41219,#41220,#41221,#41222,#41223,#41224,#41225,#41226,
#41227,#41228,#41229,#41230,#41231),.UNSPECIFIED.,.F.,.F.,(4,3,3,3,3,3,
3,3,3,3,3,3,3,3,4),(57.6741302701237,57.7622100177242,58.2601601040839,
58.7581101904436,59.2560602768033,59.754010363163,60.2519604495227,60.7499105358824,
61.2478606222421,61.7458107086018,62.2437607949614,62.7417108813211,63.2396609676808,
63.7376110540405,63.9573155773032),.UNSPECIFIED.);
#1057=B_SPLINE_CURVE_WITH_KNOTS('',3,(#41236,#41237,#41238,#41239,#41240,
#41241,#41242,#41243,#41244,#41245,#41246,#41247,#41248,#41249,#41250,#41251,
#41252,#41253,#41254,#41255,#41256,#41257,#41258,#41259,#41260,#41261,#41262,
#41263,#41264,#41265,#41266,#41267,#41268,#41269,#41270,#41271,#41272,#41273,
#41274,#41275,#41276,#41277,#41278),.UNSPECIFIED.,.F.,.F.,(4,3,3,3,3,3,
3,3,3,3,3,3,3,3,4),(-73.2079687991063,-73.1986626948747,-72.700712608515,
-72.2027625221553,-71.7048124357956,-71.206862349436,-70.7089122630762,
-70.2109621767165,-69.7130120903569,-69.2150620039972,-68.7171119176375,
-68.2191618312778,-67.7212117449181,-67.2232616585584,-66.9247834919266),
 .UNSPECIFIED.);
#1058=B_SPLINE_CURVE_WITH_KNOTS('',3,(#41279,#41280,#41281,#41282,#41283,
#41284,#41285,#41286,#41287,#41288,#41289,#41290,#41291,#41292,#41293,#41294,
#41295,#41296,#41297,#41298,#41299,#41300,#41301,#41302,#41303,#41304,#41305,
#41306,#41307,#41308,#41309,#41310,#41311,#41312,#41313,#41314,#41315,#41316,
#41317,#41318,#41319,#41320,#41321),.UNSPECIFIED.,.F.,.F.,(4,3,3,3,3,3,
3,3,3,3,3,3,3,3,4),(63.9573155773032,64.2355611404002,64.7335112267599,
65.2314613131196,65.7294113994793,66.227361485839,66.7253115721987,67.2232616585584,
67.7212117449181,68.2191618312777,68.7171119176374,69.2150620039971,69.7130120903568,
70.2109621767165,70.2405008844829),.UNSPECIFIED.);
#1059=B_SPLINE_CURVE_WITH_KNOTS('',3,(#41326,#41327,#41328,#41329,#41330,
#41331,#41332,#41333,#41334,#41335,#41336,#41337,#41338,#41339,#41340,#41341,
#41342,#41343,#41344,#41345,#41346,#41347,#41348,#41349,#41350,#41351,#41352,
#41353,#41354,#41355,#41356,#41357,#41358,#41359,#41360,#41361,#41362,#41363,
#41364,#41365),.UNSPECIFIED.,.F.,.F.,(4,3,3,3,3,3,3,3,3,3,3,3,3,4),(-79.4911541062858,
-79.174063731191,-78.6761136448313,-78.1781635584716,-77.6802134721119,
-77.1822633857523,-76.6843132993926,-76.1863632130329,-75.6884131266732,
-75.1904630403135,-74.6925129539538,-74.1945628675941,-73.6966127812344,
-73.2079687991063),.UNSPECIFIED.);
#1060=B_SPLINE_CURVE_WITH_KNOTS('',3,(#41366,#41367,#41368,#41369,#41370,
#41371,#41372,#41373,#41374,#41375,#41376,#41377,#41378,#41379,#41380,#41381,
#41382,#41383,#41384,#41385,#41386,#41387,#41388,#41389,#41390,#41391,#41392,
#41393,#41394,#41395,#41396,#41397,#41398,#41399,#41400,#41401,#41402,#41403,
#41404,#41405),.UNSPECIFIED.,.F.,.F.,(4,3,3,3,3,3,3,3,3,3,3,3,3,4),(70.2405008844829,
70.7089122630762,71.2068623494359,71.7048124357956,72.2027625221553,72.7007126085149,
73.1986626948746,73.6966127812344,74.194562867594,74.6925129539537,75.1904630403134,
75.6884131266731,76.1863632130328,76.5236861916624),.UNSPECIFIED.);
#1061=B_SPLINE_CURVE_WITH_KNOTS('',3,(#41411,#41412,#41413,#41414),
 .UNSPECIFIED.,.F.,.F.,(4,4),(91.106186954104,91.2020467387594),
 .UNSPECIFIED.);
#1062=B_SPLINE_CURVE_WITH_KNOTS('',3,(#41420,#41421,#41422,#41423,#41424,
#41425,#41426,#41427,#41428,#41429,#41430,#41431,#41432,#41433,#41434,#41435),
 .UNSPECIFIED.,.F.,.F.,(4,1,1,1,1,1,1,1,1,1,1,1,1,4),(84.8230016469245,
85.3116456290525,85.8095957154122,86.3075458017719,86.8054958881316,87.3034459744913,
87.801396060851,88.2993461472107,88.7972962335704,89.2952463199301,89.7931964062898,
90.2911464926494,90.7890965790091,91.106186954104),.UNSPECIFIED.);
#1063=B_SPLINE_CURVE_WITH_KNOTS('',3,(#41438,#41439,#41440,#41441,#41442,
#41443,#41444,#41445,#41446,#41447,#41448,#41449,#41450,#41451),
 .UNSPECIFIED.,.F.,.F.,(4,1,1,1,1,1,1,1,1,1,1,4),(84.8230016469243,84.9836287546544,
85.4815788410141,85.9795289273738,86.4774790137335,86.9754291000932,87.4733791864529,
87.9713292728126,88.4692793591723,88.967229445532,89.4651795318917,89.9631296182514),
 .UNSPECIFIED.);
#1064=B_SPLINE_CURVE_WITH_KNOTS('',3,(#41456,#41457,#41458,#41459,#41460,
#41461,#41462,#41463,#41464,#41465,#41466,#41467,#41468,#41469,#41470,#41471,
#41472),.UNSPECIFIED.,.F.,.F.,(4,1,1,1,1,1,1,1,1,1,1,1,1,1,4),(78.5398163397448,
78.8382945063765,79.3362445927362,79.8341946790959,80.3321447654556,80.8300948518153,
81.328044938175,81.8259950245347,82.3239451108944,82.8218951972541,83.3198452836138,
83.8177953699735,84.3157454563331,84.8136955426928,84.8230016469245),
 .UNSPECIFIED.);
#1065=B_SPLINE_CURVE_WITH_KNOTS('',3,(#41473,#41474,#41475,#41476,#41477,
#41478,#41479,#41480,#41481,#41482,#41483,#41484,#41485,#41486,#41487,#41488),
 .UNSPECIFIED.,.F.,.F.,(4,1,1,1,1,1,1,1,1,1,1,1,1,4),(78.5398163397448,
79.0082277183381,79.5061778046978,80.0041278910575,80.5020779774172,81.0000280637769,
81.4979781501366,81.9959282364963,82.493878322856,82.9918284092157,83.4897784955754,
83.9877285819351,84.4856786682948,84.8230016469243),.UNSPECIFIED.);
#1066=B_SPLINE_CURVE_WITH_KNOTS('',3,(#41493,#41494,#41495,#41496,#41497,
#41498,#41499,#41500,#41501,#41502,#41503,#41504,#41505,#41506,#41507,#41508,
#41509),.UNSPECIFIED.,.F.,.F.,(4,1,1,1,1,1,1,1,1,1,1,1,1,1,4),(72.2566310325653,
72.3649433837005,72.8628934700602,73.3608435564199,73.8587936427796,74.3567437291393,
74.854693815499,75.3526439018587,75.8505939882184,76.3485440745781,76.8464941609378,
77.3444442472975,77.8423943336572,78.3403444200168,78.5398163397448),
 .UNSPECIFIED.);
#1067=B_SPLINE_CURVE_WITH_KNOTS('',3,(#41510,#41511,#41512,#41513,#41514,
#41515,#41516,#41517,#41518,#41519,#41520,#41521,#41522,#41523,#41524,#41525,
#41526),.UNSPECIFIED.,.F.,.F.,(4,1,1,1,1,1,1,1,1,1,1,1,1,1,4),(72.2566310325653,
72.5348765956622,73.0328266820218,73.5307767683815,74.0287268547412,74.5266769411009,
75.0246270274606,75.5225771138203,76.02052720018,76.5184772865397,77.0164273728994,
77.5143774592591,78.0123275456188,78.5102776319785,78.5398163397448),
 .UNSPECIFIED.);
#1068=B_SPLINE_CURVE_WITH_KNOTS('',3,(#41531,#41532,#41533,#41534,#41535,
#41536,#41537,#41538,#41539,#41540,#41541,#41542,#41543,#41544,#41545,#41546),
 .UNSPECIFIED.,.F.,.F.,(4,1,1,1,1,1,1,1,1,1,1,1,1,4),(65.9734457253856,
66.3895423473842,66.8874924337439,67.3854425201036,67.8833926064633,68.381342692823,
68.8792927791827,69.3772428655424,69.8751929519021,70.3731430382618,70.8710931246215,
71.3690432109811,71.8669932973408,72.2566310325653),.UNSPECIFIED.);
#1069=B_SPLINE_CURVE_WITH_KNOTS('',3,(#41547,#41548,#41549,#41550,#41551,
#41552,#41553,#41554,#41555,#41556,#41557,#41558,#41559,#41560,#41561,#41562,
#41563),.UNSPECIFIED.,.F.,.F.,(4,1,1,1,1,1,1,1,1,1,1,1,1,1,4),(65.9734457253856,
66.0615254729862,66.5594755593459,67.0574256457055,67.5553757320652,68.0533258184249,
68.5512759047846,69.0492259911443,69.547176077504,70.0451261638637,70.5430762502234,
71.0410263365831,71.5389764229428,72.0369265093025,72.2566310325653),
 .UNSPECIFIED.);
#1070=B_SPLINE_CURVE_WITH_KNOTS('',3,(#41568,#41569,#41570,#41571,#41572,
#41573,#41574,#41575,#41576,#41577,#41578,#41579,#41580,#41581,#41582,#41583,
#41584),.UNSPECIFIED.,.F.,.F.,(4,1,1,1,1,1,1,1,1,1,1,1,1,1,4),(59.6902604182061,
59.9161912247082,60.4141413110679,60.9120913974276,61.4100414837873,61.907991570147,
62.4059416565067,62.9038917428664,63.4018418292261,63.8997919155858,64.3977420019455,
64.8956920883052,65.3936421746648,65.8915922610245,65.9734457253856),
 .UNSPECIFIED.);
#1071=B_SPLINE_CURVE_WITH_KNOTS('',3,(#41585,#41586,#41587,#41588,#41589,
#41590,#41591,#41592,#41593,#41594,#41595,#41596,#41597,#41598,#41599,#41600),
 .UNSPECIFIED.,.F.,.F.,(4,1,1,1,1,1,1,1,1,1,1,1,1,4),(59.6902604182061,
60.0861244366699,60.5840745230296,61.0820246093893,61.5799746957489,62.0779247821086,
62.5758748684683,63.073824954828,63.5717750411877,64.0697251275474,64.5676752139071,
65.0656253002668,65.5635753866265,65.9734457253856),.UNSPECIFIED.);
#1072=B_SPLINE_CURVE_WITH_KNOTS('',3,(#41605,#41606,#41607,#41608,#41609,
#41610,#41611,#41612,#41613,#41614,#41615,#41616,#41617,#41618,#41619,#41620,
#41621),.UNSPECIFIED.,.F.,.F.,(4,1,1,1,1,1,1,1,1,1,1,1,1,1,4),(53.4070751110264,
53.4428401020322,53.9407901883919,54.4387402747516,54.9366903611113,55.434640447471,
55.9325905338307,56.4305406201904,56.9284907065501,57.4264407929098,57.9243908792695,
58.4223409656292,58.9202910519889,59.4182411383485,59.6902604182061),
 .UNSPECIFIED.);
#1073=B_SPLINE_CURVE_WITH_KNOTS('',3,(#41622,#41623,#41624,#41625,#41626,
#41627,#41628,#41629,#41630,#41631,#41632,#41633,#41634,#41635,#41636,#41637,
#41638),.UNSPECIFIED.,.F.,.F.,(4,1,1,1,1,1,1,1,1,1,1,1,1,1,4),(53.4070751110264,
53.6127733139939,54.1107234003536,54.6086734867133,55.106623573073,55.6045736594326,
56.1025237457923,56.600473832152,57.0984239185117,57.5963740048714,58.0943240912311,
58.5922741775908,59.0902242639505,59.5881743503102,59.6902604182061),
 .UNSPECIFIED.);
#1074=B_SPLINE_CURVE_WITH_KNOTS('',3,(#41643,#41644,#41645,#41646,#41647,
#41648,#41649,#41650,#41651,#41652,#41653,#41654,#41655,#41656,#41657,#41658),
 .UNSPECIFIED.,.F.,.F.,(4,1,1,1,1,1,1,1,1,1,1,1,1,4),(47.1238898038469,
47.4674390657159,47.9653891520756,48.4633392384353,48.961289324795,49.4592394111547,
49.9571894975144,50.4551395838741,50.9530896702338,51.4510397565935,51.9489898429532,
52.4469399293129,52.9448900156726,53.4070751110264),.UNSPECIFIED.);
#1075=B_SPLINE_CURVE_WITH_KNOTS('',3,(#41659,#41660,#41661,#41662,#41663,
#41664,#41665,#41666,#41667,#41668,#41669,#41670,#41671,#41672,#41673,#41674,
#41675),.UNSPECIFIED.,.F.,.F.,(4,1,1,1,1,1,1,1,1,1,1,1,1,1,4),(47.1238898038469,
47.1394221913179,47.6373722776776,48.1353223640373,48.633272450397,49.1312225367567,
49.6291726231163,50.127122709476,50.6250727958357,51.1230228821954,51.6209729685551,
52.1189230549148,52.6168731412745,53.1148232276342,53.4070751110264),
 .UNSPECIFIED.);
#1076=B_SPLINE_CURVE_WITH_KNOTS('',3,(#41680,#41681,#41682,#41683,#41684,
#41685,#41686,#41687,#41688,#41689,#41690,#41691,#41692,#41693,#41694,#41695,
#41696),.UNSPECIFIED.,.F.,.F.,(4,1,1,1,1,1,1,1,1,1,1,1,1,1,4),(40.8407044966672,
40.9940879430399,41.4920380293996,41.9899881157593,42.487938202119,42.9858882884787,
43.4838383748384,43.9817884611981,44.4797385475578,44.9776886339175,45.4756387202772,
45.9735888066369,46.4715388929966,46.9694889793562,47.1238898038469),
 .UNSPECIFIED.);
#1077=B_SPLINE_CURVE_WITH_KNOTS('',3,(#41697,#41698,#41699,#41700,#41701,
#41702,#41703,#41704,#41705,#41706,#41707,#41708,#41709,#41710,#41711,#41712),
 .UNSPECIFIED.,.F.,.F.,(4,1,1,1,1,1,1,1,1,1,1,1,1,4),(40.8407044966672,
41.1640211550016,41.6619712413613,42.159921327721,42.6578714140807,43.1558215004404,
43.6537715868,44.1517216731597,44.6496717595194,45.1476218458791,45.6455719322388,
46.1435220185985,46.6414721049582,47.1238898038469),.UNSPECIFIED.);
#1078=B_SPLINE_CURVE_WITH_KNOTS('',3,(#41717,#41718,#41719,#41720,#41721,
#41722,#41723,#41724,#41725,#41726,#41727,#41728,#41729,#41730,#41731,#41732),
 .UNSPECIFIED.,.F.,.F.,(4,1,1,1,1,1,1,1,1,1,1,1,1,4),(34.5575191894877,
35.0186869067236,35.5166369930833,36.014587079443,36.5125371658027,37.0104872521624,
37.5084373385221,38.0063874248818,38.5043375112415,39.0022875976012,39.5002376839609,
39.9981877703206,40.4961378566802,40.8407044966672),.UNSPECIFIED.);
#1079=B_SPLINE_CURVE_WITH_KNOTS('',3,(#41733,#41734,#41735,#41736,#41737,
#41738,#41739,#41740,#41741,#41742,#41743,#41744,#41745,#41746,#41747,#41748,
#41749),.UNSPECIFIED.,.F.,.F.,(4,1,1,1,1,1,1,1,1,1,1,1,1,1,4),(34.5575191894877,
34.6906700323256,35.1886201186853,35.686570205045,36.1845202914047,36.6824703777644,
37.1804204641241,37.6783705504837,38.1763206368434,38.6742707232031,39.1722208095628,
39.6701708959225,40.1681209822822,40.6660710686419,40.8407044966672),
 .UNSPECIFIED.);
#1080=B_SPLINE_CURVE_WITH_KNOTS('',3,(#41754,#41755,#41756,#41757,#41758,
#41759,#41760,#41761,#41762,#41763,#41764,#41765,#41766,#41767,#41768,#41769,
#41770),.UNSPECIFIED.,.F.,.F.,(4,1,1,1,1,1,1,1,1,1,1,1,1,1,4),(28.2743338823082,
28.5453357840476,29.0432858704073,29.541235956767,30.0391860431267,30.5371361294864,
31.0350862158461,31.5330363022058,32.0309863885655,32.5289364749252,33.0268865612849,
33.5248366476446,34.0227867340043,34.520736820364,34.5575191894877),
 .UNSPECIFIED.);
#1081=B_SPLINE_CURVE_WITH_KNOTS('',3,(#41771,#41772,#41773,#41774,#41775,
#41776,#41777,#41778,#41779,#41780,#41781,#41782,#41783,#41784,#41785,#41786),
 .UNSPECIFIED.,.F.,.F.,(4,1,1,1,1,1,1,1,1,1,1,1,1,4),(28.274333882308,28.7152689960093,
29.213219082369,29.7111691687287,30.2091192550884,30.7070693414481,31.2050194278078,
31.7029695141674,32.2009196005271,32.6988696868868,33.1968197732465,33.6947698596062,
34.1927199459659,34.5575191894877),.UNSPECIFIED.);
#1082=B_SPLINE_CURVE_WITH_KNOTS('',3,(#41791,#41792,#41793,#41794,#41795,
#41796,#41797,#41798,#41799,#41800,#41801,#41802,#41803,#41804,#41805,#41806,
#41807),.UNSPECIFIED.,.F.,.F.,(4,1,1,1,1,1,1,1,1,1,1,1,1,1,4),(21.9911485751285,
22.0719846613717,22.5699347477313,23.067884834091,23.5658349204507,24.0637850068104,
24.5617350931701,25.0596851795298,25.5576352658895,26.0555853522492,26.5535354386089,
27.0514855249686,27.5494356113283,28.047385697688,28.2743338823082),
 .UNSPECIFIED.);
#1083=B_SPLINE_CURVE_WITH_KNOTS('',3,(#41808,#41809,#41810,#41811,#41812,
#41813,#41814,#41815,#41816,#41817,#41818,#41819,#41820,#41821,#41822,#41823,
#41824),.UNSPECIFIED.,.F.,.F.,(4,1,1,1,1,1,1,1,1,1,1,1,1,1,4),(21.9911485751285,
22.2419178733333,22.739867959693,23.2378180460527,23.7357681324124,24.2337182187721,
24.7316683051318,25.2296183914915,25.7275684778511,26.2255185642108,26.7234686505705,
27.2214187369302,27.7193688232899,28.2173189096496,28.274333882308),
 .UNSPECIFIED.);
#1084=B_SPLINE_CURVE_WITH_KNOTS('',3,(#41829,#41830,#41831,#41832,#41833,
#41834,#41835,#41836,#41837,#41838,#41839,#41840,#41841,#41842,#41843,#41844),
 .UNSPECIFIED.,.F.,.F.,(4,1,1,1,1,1,1,1,1,1,1,1,1,4),(15.707963267949,16.0965836250554,
16.594533711415,17.0924837977747,17.5904338841344,18.0883839704941,18.5863340568538,
19.0842841432135,19.5822342295732,20.0801843159329,20.5781344022926,21.0760844886523,
21.574034575012,21.9911485751285),.UNSPECIFIED.);
#1085=B_SPLINE_CURVE_WITH_KNOTS('',3,(#41845,#41846,#41847,#41848,#41849,
#41850,#41851,#41852,#41853,#41854,#41855,#41856,#41857,#41858,#41859,#41860,
#41861),.UNSPECIFIED.,.F.,.F.,(4,1,1,1,1,1,1,1,1,1,1,1,1,1,4),(15.707963267949,
15.7685667506573,16.266516837017,16.7644669233767,17.2624170097364,17.7603670960961,
18.2583171824558,18.7562672688155,19.2542173551752,19.7521674415349,20.2501175278945,
20.7480676142542,21.2460177006139,21.7439677869736,21.9911485751285),
 .UNSPECIFIED.);
#1086=B_SPLINE_CURVE_WITH_KNOTS('',3,(#41864,#41865,#41866,#41867,#41868,
#41869,#41870,#41871,#41872,#41873,#41874,#41875,#41876,#41877,#41878,#41879,
#41880,#41881,#41882,#41883,#41884,#41885,#41886,#41887,#41888,#41889,#41890,
#41891,#41892,#41893,#41894,#41895,#41896,#41897,#41898,#41899,#41900,#41901,
#41902,#41903,#41904,#41905,#41906,#41907,#41908,#41909,#41910,#41911,#41912,
#41913,#41914,#41915,#41916,#41917,#41918,#41919,#41920,#41921,#41922,#41923,
#41924,#41925,#41926,#41927,#41928,#41929,#41930,#41931,#41932,#41933,#41934,
#41935,#41936,#41937,#41938,#41939,#41940,#41941,#41942),.UNSPECIFIED.,
 .F.,.F.,(4,3,3,3,3,3,3,3,3,3,3,3,3,3,3,3,3,3,3,3,3,3,3,3,3,3,4),(-2.30573780455543,
-2.21841113392645,-2.08749160267076,-2.03463636793378,-2.00263204080081,
-1.86521061460393,-1.77569625734445,-1.73401588570404,-1.69473300890369,
-1.55556413645857,-1.41514237879565,-1.33427014934624,-1.30800108531491,
-1.16478112610678,-1.14989664424401,-1.00863390696719,-0.941358480514188,
-0.905079352339792,-0.875958582765696,-0.729465446527128,-0.584845695136702,
-0.511739983244614,-0.464615362770142,-0.437368675712909,-0.289286735155622,
-0.139857796807127,0.),.UNSPECIFIED.);
#1087=B_SPLINE_CURVE_WITH_KNOTS('',3,(#41947,#41948,#41949,#41950,#41951,
#41952,#41953,#41954,#41955,#41956,#41957,#41958,#41959,#41960,#41961,#41962,
#41963,#41964,#41965,#41966,#41967,#41968,#41969,#41970,#41971,#41972,#41973,
#41974,#41975,#41976,#41977,#41978,#41979,#41980,#41981,#41982,#41983,#41984,
#41985,#41986,#41987,#41988,#41989,#41990,#41991,#41992,#41993,#41994,#41995,
#41996,#41997,#41998,#41999,#42000,#42001,#42002,#42003,#42004,#42005,#42006,
#42007,#42008,#42009,#42010,#42011,#42012,#42013,#42014,#42015,#42016,#42017,
#42018,#42019,#42020,#42021,#42022,#42023,#42024,#42025,#42026,#42027,#42028),
 .UNSPECIFIED.,.F.,.F.,(4,3,3,3,3,3,3,3,3,3,3,3,3,3,3,3,3,3,3,3,3,3,3,3,
3,3,3,4),(-2.29817876007981,-2.19741091509423,-2.05273312368805,-1.99504166905861,
-1.96232249553947,-1.81492097586906,-1.71681036266927,-1.68268796625865,
-1.65188428124604,-1.61869974946949,-1.47364208734527,-1.32963263754991,
-1.25161162956993,-1.22444539494046,-1.08298576005188,-1.05905266124946,
-0.924129685546555,-0.862356703818927,-0.817065087590977,-0.790581206788844,
-0.652351590986891,-0.519360758437836,-0.454238466605207,-0.402777609553242,
-0.376224313666366,-0.240439074152116,-0.107056245968069,0.),
 .UNSPECIFIED.);
#1088=B_SPLINE_CURVE_WITH_KNOTS('',3,(#42697,#42698,#42699,#42700,#42701,
#42702,#42703,#42704,#42705,#42706,#42707,#42708,#42709,#42710,#42711,#42712,
#42713,#42714,#42715,#42716,#42717,#42718),.UNSPECIFIED.,.F.,.F.,(4,3,3,
3,3,3,3,4),(76.5236861916624,76.6843132993925,77.1822633857522,77.6802134721119,
78.1781635584716,78.6761136448312,79.1740637311909,79.5870138909412),
 .UNSPECIFIED.);
#1089=B_SPLINE_CURVE_WITH_KNOTS('',3,(#42720,#42721,#42722,#42723,#42724,
#42725,#42726,#42727,#42728,#42729,#42730,#42731,#42732,#42733,#42734,#42735,
#42736,#42737,#42738,#42739,#42740,#42741,#42742,#42743,#42744,#42745,#42746,
#42747,#42748,#42749,#42750,#42751,#42752,#42753,#42754,#42755,#42756,#42757,
#42758,#42759,#42760,#42761,#42762,#42763,#42764,#42765,#42766,#42767,#42768,
#42769,#42770,#42771,#42772,#42773,#42774,#42775,#42776,#42777,#42778,#42779,
#42780,#42781,#42782,#42783,#42784,#42785,#42786,#42787,#42788,#42789,#42790,
#42791,#42792,#42793,#42794,#42795,#42796,#42797,#42798),.UNSPECIFIED.,
 .F.,.F.,(4,3,3,3,3,3,3,3,3,3,3,3,3,3,3,3,3,3,3,3,3,3,3,3,3,3,4),(-2.30573780455542,
-2.2184111339264,-2.08749160267071,-2.03463636764165,-2.00263204069499,
-1.86521061414297,-1.77569625699512,-1.73401588567174,-1.69473300890364,
-1.555564136972,-1.41514237955304,-1.33427015017412,-1.3080010854375,-1.16478112641558,
-1.14989664424397,-1.00863390696714,-0.94135847965341,-0.905079350045409,
-0.875958582289399,-0.729465445933032,-0.584845695136671,-0.511739983244587,
-0.464615363394834,-0.437368676240646,-0.289286726941639,-0.139857794152545,
0.),.UNSPECIFIED.);
#1090=B_SPLINE_CURVE_WITH_KNOTS('',3,(#42799,#42800,#42801,#42802,#42803,
#42804,#42805,#42806,#42807,#42808,#42809,#42810,#42811,#42812),
 .UNSPECIFIED.,.F.,.F.,(4,1,1,1,1,1,1,1,1,1,1,4),(10.3761157273102,10.7890658870604,
11.2870159734201,11.7849660597798,12.2829161461395,12.7808662324992,13.2788163188589,
13.7767664052186,14.2747164915782,14.7726665779379,15.2706166642976,15.707963267949),
 .UNSPECIFIED.);
#1091=B_SPLINE_CURVE_WITH_KNOTS('',3,(#42818,#42819,#42820,#42821,#42822,
#42823,#42824,#42825,#42826,#42827,#42828,#42829,#42830,#42831,#42832,#42833,
#42834,#42835,#42836,#42837,#42838,#42839,#42840,#42841,#42842,#42843,#42844,
#42845,#42846,#42847,#42848,#42849,#42850,#42851,#42852,#42853,#42854,#42855,
#42856,#42857,#42858,#42859,#42860,#42861,#42862,#42863,#42864,#42865,#42866,
#42867,#42868,#42869,#42870,#42871,#42872,#42873,#42874,#42875,#42876,#42877,
#42878,#42879,#42880,#42881,#42882,#42883,#42884,#42885,#42886,#42887,#42888,
#42889,#42890,#42891,#42892,#42893,#42894,#42895,#42896,#42897,#42898,#42899),
 .UNSPECIFIED.,.F.,.F.,(4,3,3,3,3,3,3,3,3,3,3,3,3,3,3,3,3,3,3,3,3,3,3,3,
3,3,3,4),(-2.29817876007991,-2.19741091509428,-2.05273312368808,-1.99504166925756,
-1.96232249570202,-1.81492097587876,-1.71681036267412,-1.68268796661413,
-1.6518842813445,-1.61869974946948,-1.47364208662842,-1.32963263430615,
-1.25161162484676,-1.22444539341282,-1.08298575668718,-1.05905266124945,
-0.924129685546546,-0.862356703698319,-0.817065087328252,-0.790581206971903,
-0.652351598429523,-0.519360758437847,-0.454238469053417,-0.40277761002181,
-0.37622431360753,-0.240439072833657,-0.107056229103949,0.),
 .UNSPECIFIED.);
#1092=B_SPLINE_CURVE_WITH_KNOTS('',3,(#42902,#42903,#42904,#42905,#42906,
#42907,#42908,#42909,#42910,#42911,#42912,#42913),.UNSPECIFIED.,.F.,.F.,
(4,1,1,1,1,1,1,1,1,4),(11.6150328478181,12.1129829341778,12.6109330205375,
13.1088831068972,13.6068331932569,14.1047832796166,14.6027333659763,15.100683452336,
15.5986335386957,15.707963267949),.UNSPECIFIED.);
#1093=B_SPLINE_CURVE_WITH_KNOTS('',3,(#43582,#43583,#43584,#43585,#43586,
#43587,#43588,#43589,#43590,#43591,#43592,#43593,#43594,#43595,#43596,#43597),
 .UNSPECIFIED.,.F.,.F.,(4,3,3,3,3,4),(-81.6638141629894,-81.1658640766298,
-80.6679139902701,-80.1699639039104,-79.6720138175507,-79.4911541062858),
 .UNSPECIFIED.);
#1722=PLANE('',#27261);
#1723=PLANE('',#27264);
#1724=PLANE('',#27271);
#1725=PLANE('',#27277);
#1726=PLANE('',#27282);
#2694=FACE_OUTER_BOUND('',#4187,.T.);
#2695=FACE_OUTER_BOUND('',#4188,.T.);
#2696=FACE_OUTER_BOUND('',#4189,.T.);
#2697=FACE_OUTER_BOUND('',#4190,.T.);
#2698=FACE_OUTER_BOUND('',#4191,.T.);
#2699=FACE_OUTER_BOUND('',#4192,.T.);
#2700=FACE_OUTER_BOUND('',#4193,.T.);
#2701=FACE_OUTER_BOUND('',#4194,.T.);
#2702=FACE_OUTER_BOUND('',#4195,.T.);
#2703=FACE_OUTER_BOUND('',#4196,.T.);
#2704=FACE_OUTER_BOUND('',#4197,.T.);
#2705=FACE_OUTER_BOUND('',#4198,.T.);
#2706=FACE_OUTER_BOUND('',#4199,.T.);
#2707=FACE_OUTER_BOUND('',#4200,.T.);
#2708=FACE_OUTER_BOUND('',#4201,.T.);
#2709=FACE_OUTER_BOUND('',#4202,.T.);
#2710=FACE_OUTER_BOUND('',#4203,.T.);
#2711=FACE_OUTER_BOUND('',#4204,.T.);
#2712=FACE_OUTER_BOUND('',#4205,.T.);
#2713=FACE_OUTER_BOUND('',#4206,.T.);
#2714=FACE_OUTER_BOUND('',#4207,.T.);
#2715=FACE_OUTER_BOUND('',#4208,.T.);
#2716=FACE_OUTER_BOUND('',#4209,.T.);
#2717=FACE_OUTER_BOUND('',#4210,.T.);
#2718=FACE_OUTER_BOUND('',#4211,.T.);
#2719=FACE_OUTER_BOUND('',#4212,.T.);
#2720=FACE_OUTER_BOUND('',#4213,.T.);
#2721=FACE_OUTER_BOUND('',#4214,.T.);
#2722=FACE_OUTER_BOUND('',#4215,.T.);
#2723=FACE_OUTER_BOUND('',#4216,.T.);
#2724=FACE_OUTER_BOUND('',#4217,.T.);
#2725=FACE_OUTER_BOUND('',#4218,.T.);
#2726=FACE_OUTER_BOUND('',#4219,.T.);
#2727=FACE_OUTER_BOUND('',#4220,.T.);
#2728=FACE_OUTER_BOUND('',#4221,.T.);
#2729=FACE_OUTER_BOUND('',#4222,.T.);
#2730=FACE_OUTER_BOUND('',#4224,.T.);
#2731=FACE_OUTER_BOUND('',#4225,.T.);
#2732=FACE_OUTER_BOUND('',#4226,.T.);
#4187=EDGE_LOOP('',(#18198,#18199,#18200,#18201));
#4188=EDGE_LOOP('',(#18202,#18203,#18204,#18205));
#4189=EDGE_LOOP('',(#18206,#18207,#18208,#18209));
#4190=EDGE_LOOP('',(#18210,#18211,#18212,#18213));
#4191=EDGE_LOOP('',(#18214,#18215,#18216,#18217));
#4192=EDGE_LOOP('',(#18218,#18219,#18220,#18221));
#4193=EDGE_LOOP('',(#18222,#18223,#18224,#18225));
#4194=EDGE_LOOP('',(#18226,#18227,#18228,#18229));
#4195=EDGE_LOOP('',(#18230,#18231,#18232,#18233));
#4196=EDGE_LOOP('',(#18234,#18235,#18236,#18237));
#4197=EDGE_LOOP('',(#18238,#18239,#18240,#18241));
#4198=EDGE_LOOP('',(#18242,#18243,#18244,#18245));
#4199=EDGE_LOOP('',(#18246,#18247,#18248,#18249));
#4200=EDGE_LOOP('',(#18250,#18251,#18252));
#4201=EDGE_LOOP('',(#18253,#18254,#18255,#18256,#18257));
#4202=EDGE_LOOP('',(#18258,#18259,#18260,#18261));
#4203=EDGE_LOOP('',(#18262,#18263,#18264,#18265));
#4204=EDGE_LOOP('',(#18266,#18267,#18268,#18269));
#4205=EDGE_LOOP('',(#18270,#18271,#18272,#18273));
#4206=EDGE_LOOP('',(#18274,#18275,#18276,#18277));
#4207=EDGE_LOOP('',(#18278,#18279,#18280,#18281));
#4208=EDGE_LOOP('',(#18282,#18283,#18284,#18285));
#4209=EDGE_LOOP('',(#18286,#18287,#18288,#18289));
#4210=EDGE_LOOP('',(#18290,#18291,#18292,#18293));
#4211=EDGE_LOOP('',(#18294,#18295,#18296,#18297));
#4212=EDGE_LOOP('',(#18298,#18299,#18300,#18301));
#4213=EDGE_LOOP('',(#18302,#18303,#18304,#18305,#18306,#18307));
#4214=EDGE_LOOP('',(#18308,#18309,#18310,#18311,#18312,#18313,#18314,#18315,
#18316,#18317,#18318,#18319,#18320,#18321,#18322,#18323,#18324,#18325,#18326,
#18327,#18328,#18329,#18330,#18331,#18332,#18333,#18334,#18335,#18336));
#4215=EDGE_LOOP('',(#18337,#18338,#18339,#18340,#18341));
#4216=EDGE_LOOP('',(#18342,#18343,#18344,#18345));
#4217=EDGE_LOOP('',(#18346,#18347,#18348,#18349,#18350,#18351,#18352,#18353,
#18354,#18355,#18356,#18357,#18358,#18359,#18360,#18361,#18362,#18363,#18364,
#18365,#18366,#18367,#18368,#18369,#18370,#18371,#18372,#18373,#18374,#18375));
#4218=EDGE_LOOP('',(#18376,#18377,#18378,#18379));
#4219=EDGE_LOOP('',(#18380));
#4220=EDGE_LOOP('',(#18381,#18382,#18383,#18384));
#4221=EDGE_LOOP('',(#18385,#18386,#18387,#18388));
#4222=EDGE_LOOP('',(#18389));
#4223=EDGE_LOOP('',(#18390));
#4224=EDGE_LOOP('',(#18391,#18392,#18393,#18394,#18395,#18396));
#4225=EDGE_LOOP('',(#18397,#18398,#18399,#18400,#18401,#18402));
#4226=EDGE_LOOP('',(#18403));
#5784=LINE('',#40326,#8281);
#5785=LINE('',#40359,#8282);
#5786=LINE('',#40443,#8283);
#5787=LINE('',#40533,#8284);
#5788=LINE('',#40623,#8285);
#5789=LINE('',#40707,#8286);
#5790=LINE('',#40797,#8287);
#5791=LINE('',#40881,#8288);
#5792=LINE('',#40971,#8289);
#5793=LINE('',#41061,#8290);
#5794=LINE('',#41145,#8291);
#5795=LINE('',#41235,#8292);
#5796=LINE('',#41325,#8293);
#5797=LINE('',#41409,#8294);
#5798=LINE('',#41419,#8295);
#5799=LINE('',#41455,#8296);
#5800=LINE('',#41492,#8297);
#5801=LINE('',#41530,#8298);
#5802=LINE('',#41567,#8299);
#5803=LINE('',#41604,#8300);
#5804=LINE('',#41642,#8301);
#5805=LINE('',#41679,#8302);
#5806=LINE('',#41716,#8303);
#5807=LINE('',#41753,#8304);
#5808=LINE('',#41790,#8305);
#5809=LINE('',#41828,#8306);
#5810=LINE('',#43606,#8307);
#5811=LINE('',#43610,#8308);
#5812=LINE('',#43615,#8309);
#5813=LINE('',#43619,#8310);
#8281=VECTOR('',#29499,1.2);
#8282=VECTOR('',#29504,1.2);
#8283=VECTOR('',#29507,1.2);
#8284=VECTOR('',#29510,1.2);
#8285=VECTOR('',#29513,1.2);
#8286=VECTOR('',#29516,1.2);
#8287=VECTOR('',#29519,1.2);
#8288=VECTOR('',#29522,1.2);
#8289=VECTOR('',#29525,1.2);
#8290=VECTOR('',#29528,1.2);
#8291=VECTOR('',#29531,1.2);
#8292=VECTOR('',#29534,1.2);
#8293=VECTOR('',#29537,1.2);
#8294=VECTOR('',#29540,1.016475);
#8295=VECTOR('',#29545,1.016475);
#8296=VECTOR('',#29550,1.016475);
#8297=VECTOR('',#29553,1.016475);
#8298=VECTOR('',#29556,1.016475);
#8299=VECTOR('',#29559,1.016475);
#8300=VECTOR('',#29562,1.016475);
#8301=VECTOR('',#29565,1.016475);
#8302=VECTOR('',#29568,1.016475);
#8303=VECTOR('',#29571,1.016475);
#8304=VECTOR('',#29574,1.016475);
#8305=VECTOR('',#29577,1.016475);
#8306=VECTOR('',#29580,1.016475);
#8307=VECTOR('',#29609,1.85);
#8308=VECTOR('',#29614,2.);
#8309=VECTOR('',#29621,1.225);
#8310=VECTOR('',#29626,1.125);
#10712=CIRCLE('',#27233,1.188225);
#10713=CIRCLE('',#27247,1.016475);
#10714=CIRCLE('',#27249,1.016475);
#10715=CIRCLE('',#27262,1.188225);
#10716=CIRCLE('',#27263,1.188225);
#10717=CIRCLE('',#27265,1.188225);
#10718=CIRCLE('',#27266,1.188225);
#10719=CIRCLE('',#27267,1.016475);
#10720=CIRCLE('',#27270,1.188225);
#10721=CIRCLE('',#27272,1.7);
#10722=CIRCLE('',#27274,2.);
#10723=CIRCLE('',#27276,2.);
#10724=CIRCLE('',#27278,1.25);
#10725=CIRCLE('',#27281,1.05);
#11371=VERTEX_POINT('',#40324);
#11372=VERTEX_POINT('',#40325);
#11373=VERTEX_POINT('',#40327);
#11374=VERTEX_POINT('',#40344);
#11375=VERTEX_POINT('',#40357);
#11376=VERTEX_POINT('',#40358);
#11377=VERTEX_POINT('',#40441);
#11378=VERTEX_POINT('',#40442);
#11379=VERTEX_POINT('',#40531);
#11380=VERTEX_POINT('',#40532);
#11381=VERTEX_POINT('',#40621);
#11382=VERTEX_POINT('',#40622);
#11383=VERTEX_POINT('',#40705);
#11384=VERTEX_POINT('',#40706);
#11385=VERTEX_POINT('',#40795);
#11386=VERTEX_POINT('',#40796);
#11387=VERTEX_POINT('',#40879);
#11388=VERTEX_POINT('',#40880);
#11389=VERTEX_POINT('',#40969);
#11390=VERTEX_POINT('',#40970);
#11391=VERTEX_POINT('',#41059);
#11392=VERTEX_POINT('',#41060);
#11393=VERTEX_POINT('',#41143);
#11394=VERTEX_POINT('',#41144);
#11395=VERTEX_POINT('',#41233);
#11396=VERTEX_POINT('',#41234);
#11397=VERTEX_POINT('',#41323);
#11398=VERTEX_POINT('',#41324);
#11399=VERTEX_POINT('',#41407);
#11400=VERTEX_POINT('',#41408);
#11401=VERTEX_POINT('',#41410);
#11402=VERTEX_POINT('',#41417);
#11403=VERTEX_POINT('',#41418);
#11404=VERTEX_POINT('',#41436);
#11405=VERTEX_POINT('',#41453);
#11406=VERTEX_POINT('',#41454);
#11407=VERTEX_POINT('',#41490);
#11408=VERTEX_POINT('',#41491);
#11409=VERTEX_POINT('',#41528);
#11410=VERTEX_POINT('',#41529);
#11411=VERTEX_POINT('',#41565);
#11412=VERTEX_POINT('',#41566);
#11413=VERTEX_POINT('',#41602);
#11414=VERTEX_POINT('',#41603);
#11415=VERTEX_POINT('',#41640);
#11416=VERTEX_POINT('',#41641);
#11417=VERTEX_POINT('',#41677);
#11418=VERTEX_POINT('',#41678);
#11419=VERTEX_POINT('',#41714);
#11420=VERTEX_POINT('',#41715);
#11421=VERTEX_POINT('',#41751);
#11422=VERTEX_POINT('',#41752);
#11423=VERTEX_POINT('',#41788);
#11424=VERTEX_POINT('',#41789);
#11425=VERTEX_POINT('',#41826);
#11426=VERTEX_POINT('',#41827);
#11427=VERTEX_POINT('',#41863);
#11428=VERTEX_POINT('',#41943);
#11429=VERTEX_POINT('',#41945);
#11430=VERTEX_POINT('',#42719);
#11431=VERTEX_POINT('',#42814);
#11432=VERTEX_POINT('',#42817);
#11433=VERTEX_POINT('',#43601);
#11434=VERTEX_POINT('',#43604);
#11435=VERTEX_POINT('',#43608);
#11436=VERTEX_POINT('',#43612);
#11437=VERTEX_POINT('',#43617);
#13952=EDGE_CURVE('',#11371,#11372,#5784,.T.);
#13953=EDGE_CURVE('',#11371,#11373,#1035,.T.);
#13954=EDGE_CURVE('',#11373,#11374,#10712,.F.);
#13955=EDGE_CURVE('',#11374,#11372,#1036,.T.);
#13956=EDGE_CURVE('',#11375,#11376,#5785,.T.);
#13957=EDGE_CURVE('',#11375,#11371,#1037,.T.);
#13958=EDGE_CURVE('',#11372,#11376,#1038,.T.);
#13959=EDGE_CURVE('',#11377,#11378,#5786,.T.);
#13960=EDGE_CURVE('',#11377,#11375,#1039,.T.);
#13961=EDGE_CURVE('',#11376,#11378,#1040,.T.);
#13962=EDGE_CURVE('',#11379,#11380,#5787,.T.);
#13963=EDGE_CURVE('',#11379,#11377,#1041,.T.);
#13964=EDGE_CURVE('',#11378,#11380,#1042,.T.);
#13965=EDGE_CURVE('',#11381,#11382,#5788,.T.);
#13966=EDGE_CURVE('',#11381,#11379,#1043,.T.);
#13967=EDGE_CURVE('',#11380,#11382,#1044,.T.);
#13968=EDGE_CURVE('',#11383,#11384,#5789,.T.);
#13969=EDGE_CURVE('',#11383,#11381,#1045,.T.);
#13970=EDGE_CURVE('',#11382,#11384,#1046,.T.);
#13971=EDGE_CURVE('',#11385,#11386,#5790,.T.);
#13972=EDGE_CURVE('',#11385,#11383,#1047,.T.);
#13973=EDGE_CURVE('',#11384,#11386,#1048,.T.);
#13974=EDGE_CURVE('',#11387,#11388,#5791,.T.);
#13975=EDGE_CURVE('',#11387,#11385,#1049,.T.);
#13976=EDGE_CURVE('',#11386,#11388,#1050,.T.);
#13977=EDGE_CURVE('',#11389,#11390,#5792,.T.);
#13978=EDGE_CURVE('',#11389,#11387,#1051,.T.);
#13979=EDGE_CURVE('',#11388,#11390,#1052,.T.);
#13980=EDGE_CURVE('',#11391,#11392,#5793,.T.);
#13981=EDGE_CURVE('',#11391,#11389,#1053,.T.);
#13982=EDGE_CURVE('',#11390,#11392,#1054,.T.);
#13983=EDGE_CURVE('',#11393,#11394,#5794,.T.);
#13984=EDGE_CURVE('',#11393,#11391,#1055,.T.);
#13985=EDGE_CURVE('',#11392,#11394,#1056,.T.);
#13986=EDGE_CURVE('',#11395,#11396,#5795,.T.);
#13987=EDGE_CURVE('',#11395,#11393,#1057,.T.);
#13988=EDGE_CURVE('',#11394,#11396,#1058,.T.);
#13989=EDGE_CURVE('',#11397,#11398,#5796,.T.);
#13990=EDGE_CURVE('',#11397,#11395,#1059,.T.);
#13991=EDGE_CURVE('',#11396,#11398,#1060,.T.);
#13992=EDGE_CURVE('',#11399,#11400,#5797,.T.);
#13993=EDGE_CURVE('',#11399,#11401,#1061,.T.);
#13994=EDGE_CURVE('',#11400,#11401,#10713,.T.);
#13995=EDGE_CURVE('',#11402,#11403,#5798,.T.);
#13996=EDGE_CURVE('',#11402,#11399,#1062,.T.);
#13997=EDGE_CURVE('',#11404,#11400,#10714,.T.);
#13998=EDGE_CURVE('',#11403,#11404,#1063,.T.);
#13999=EDGE_CURVE('',#11405,#11406,#5799,.T.);
#14000=EDGE_CURVE('',#11405,#11402,#1064,.T.);
#14001=EDGE_CURVE('',#11406,#11403,#1065,.T.);
#14002=EDGE_CURVE('',#11407,#11408,#5800,.T.);
#14003=EDGE_CURVE('',#11407,#11405,#1066,.T.);
#14004=EDGE_CURVE('',#11408,#11406,#1067,.T.);
#14005=EDGE_CURVE('',#11409,#11410,#5801,.T.);
#14006=EDGE_CURVE('',#11409,#11407,#1068,.T.);
#14007=EDGE_CURVE('',#11410,#11408,#1069,.T.);
#14008=EDGE_CURVE('',#11411,#11412,#5802,.T.);
#14009=EDGE_CURVE('',#11411,#11409,#1070,.T.);
#14010=EDGE_CURVE('',#11412,#11410,#1071,.T.);
#14011=EDGE_CURVE('',#11413,#11414,#5803,.T.);
#14012=EDGE_CURVE('',#11413,#11411,#1072,.T.);
#14013=EDGE_CURVE('',#11414,#11412,#1073,.T.);
#14014=EDGE_CURVE('',#11415,#11416,#5804,.T.);
#14015=EDGE_CURVE('',#11415,#11413,#1074,.T.);
#14016=EDGE_CURVE('',#11416,#11414,#1075,.T.);
#14017=EDGE_CURVE('',#11417,#11418,#5805,.T.);
#14018=EDGE_CURVE('',#11417,#11415,#1076,.T.);
#14019=EDGE_CURVE('',#11418,#11416,#1077,.T.);
#14020=EDGE_CURVE('',#11419,#11420,#5806,.T.);
#14021=EDGE_CURVE('',#11419,#11417,#1078,.T.);
#14022=EDGE_CURVE('',#11420,#11418,#1079,.T.);
#14023=EDGE_CURVE('',#11421,#11422,#5807,.T.);
#14024=EDGE_CURVE('',#11421,#11419,#1080,.T.);
#14025=EDGE_CURVE('',#11422,#11420,#1081,.T.);
#14026=EDGE_CURVE('',#11423,#11424,#5808,.T.);
#14027=EDGE_CURVE('',#11423,#11421,#1082,.T.);
#14028=EDGE_CURVE('',#11424,#11422,#1083,.T.);
#14029=EDGE_CURVE('',#11425,#11426,#5809,.T.);
#14030=EDGE_CURVE('',#11425,#11423,#1084,.T.);
#14031=EDGE_CURVE('',#11426,#11424,#1085,.T.);
#14032=EDGE_CURVE('',#11401,#11427,#1086,.T.);
#14033=EDGE_CURVE('',#11428,#11427,#10715,.F.);
#14034=EDGE_CURVE('',#11429,#11428,#10716,.F.);
#14035=EDGE_CURVE('',#11429,#11404,#1087,.T.);
#14036=EDGE_CURVE('',#11398,#11429,#1088,.T.);
#14037=EDGE_CURVE('',#11430,#11374,#1089,.T.);
#14038=EDGE_CURVE('',#11430,#11426,#1090,.T.);
#14039=EDGE_CURVE('',#11374,#11431,#10717,.F.);
#14040=EDGE_CURVE('',#11431,#11373,#10718,.F.);
#14041=EDGE_CURVE('',#11373,#11432,#1091,.T.);
#14042=EDGE_CURVE('',#11432,#11430,#10719,.T.);
#14043=EDGE_CURVE('',#11432,#11425,#1092,.T.);
#14044=EDGE_CURVE('',#11427,#11397,#1093,.T.);
#14045=EDGE_CURVE('',#11427,#11429,#10720,.F.);
#14046=EDGE_CURVE('',#11433,#11433,#10721,.T.);
#14047=EDGE_CURVE('',#11434,#11434,#10722,.T.);
#14048=EDGE_CURVE('',#11434,#11433,#5810,.T.);
#14049=EDGE_CURVE('',#11435,#11435,#10723,.T.);
#14050=EDGE_CURVE('',#11435,#11434,#5811,.T.);
#14051=EDGE_CURVE('',#11436,#11436,#10724,.T.);
#14052=EDGE_CURVE('',#11431,#11436,#5812,.T.);
#14053=EDGE_CURVE('',#11437,#11437,#10725,.T.);
#14054=EDGE_CURVE('',#11437,#11428,#5813,.T.);
#18198=ORIENTED_EDGE('',*,*,#13952,.F.);
#18199=ORIENTED_EDGE('',*,*,#13953,.T.);
#18200=ORIENTED_EDGE('',*,*,#13954,.T.);
#18201=ORIENTED_EDGE('',*,*,#13955,.T.);
#18202=ORIENTED_EDGE('',*,*,#13956,.F.);
#18203=ORIENTED_EDGE('',*,*,#13957,.T.);
#18204=ORIENTED_EDGE('',*,*,#13952,.T.);
#18205=ORIENTED_EDGE('',*,*,#13958,.T.);
#18206=ORIENTED_EDGE('',*,*,#13959,.F.);
#18207=ORIENTED_EDGE('',*,*,#13960,.T.);
#18208=ORIENTED_EDGE('',*,*,#13956,.T.);
#18209=ORIENTED_EDGE('',*,*,#13961,.T.);
#18210=ORIENTED_EDGE('',*,*,#13962,.F.);
#18211=ORIENTED_EDGE('',*,*,#13963,.T.);
#18212=ORIENTED_EDGE('',*,*,#13959,.T.);
#18213=ORIENTED_EDGE('',*,*,#13964,.T.);
#18214=ORIENTED_EDGE('',*,*,#13965,.F.);
#18215=ORIENTED_EDGE('',*,*,#13966,.T.);
#18216=ORIENTED_EDGE('',*,*,#13962,.T.);
#18217=ORIENTED_EDGE('',*,*,#13967,.T.);
#18218=ORIENTED_EDGE('',*,*,#13968,.F.);
#18219=ORIENTED_EDGE('',*,*,#13969,.T.);
#18220=ORIENTED_EDGE('',*,*,#13965,.T.);
#18221=ORIENTED_EDGE('',*,*,#13970,.T.);
#18222=ORIENTED_EDGE('',*,*,#13971,.F.);
#18223=ORIENTED_EDGE('',*,*,#13972,.T.);
#18224=ORIENTED_EDGE('',*,*,#13968,.T.);
#18225=ORIENTED_EDGE('',*,*,#13973,.T.);
#18226=ORIENTED_EDGE('',*,*,#13974,.F.);
#18227=ORIENTED_EDGE('',*,*,#13975,.T.);
#18228=ORIENTED_EDGE('',*,*,#13971,.T.);
#18229=ORIENTED_EDGE('',*,*,#13976,.T.);
#18230=ORIENTED_EDGE('',*,*,#13977,.F.);
#18231=ORIENTED_EDGE('',*,*,#13978,.T.);
#18232=ORIENTED_EDGE('',*,*,#13974,.T.);
#18233=ORIENTED_EDGE('',*,*,#13979,.T.);
#18234=ORIENTED_EDGE('',*,*,#13980,.F.);
#18235=ORIENTED_EDGE('',*,*,#13981,.T.);
#18236=ORIENTED_EDGE('',*,*,#13977,.T.);
#18237=ORIENTED_EDGE('',*,*,#13982,.T.);
#18238=ORIENTED_EDGE('',*,*,#13983,.F.);
#18239=ORIENTED_EDGE('',*,*,#13984,.T.);
#18240=ORIENTED_EDGE('',*,*,#13980,.T.);
#18241=ORIENTED_EDGE('',*,*,#13985,.T.);
#18242=ORIENTED_EDGE('',*,*,#13986,.F.);
#18243=ORIENTED_EDGE('',*,*,#13987,.T.);
#18244=ORIENTED_EDGE('',*,*,#13983,.T.);
#18245=ORIENTED_EDGE('',*,*,#13988,.T.);
#18246=ORIENTED_EDGE('',*,*,#13989,.F.);
#18247=ORIENTED_EDGE('',*,*,#13990,.T.);
#18248=ORIENTED_EDGE('',*,*,#13986,.T.);
#18249=ORIENTED_EDGE('',*,*,#13991,.T.);
#18250=ORIENTED_EDGE('',*,*,#13992,.F.);
#18251=ORIENTED_EDGE('',*,*,#13993,.T.);
#18252=ORIENTED_EDGE('',*,*,#13994,.F.);
#18253=ORIENTED_EDGE('',*,*,#13995,.F.);
#18254=ORIENTED_EDGE('',*,*,#13996,.T.);
#18255=ORIENTED_EDGE('',*,*,#13992,.T.);
#18256=ORIENTED_EDGE('',*,*,#13997,.F.);
#18257=ORIENTED_EDGE('',*,*,#13998,.F.);
#18258=ORIENTED_EDGE('',*,*,#13999,.F.);
#18259=ORIENTED_EDGE('',*,*,#14000,.T.);
#18260=ORIENTED_EDGE('',*,*,#13995,.T.);
#18261=ORIENTED_EDGE('',*,*,#14001,.F.);
#18262=ORIENTED_EDGE('',*,*,#14002,.F.);
#18263=ORIENTED_EDGE('',*,*,#14003,.T.);
#18264=ORIENTED_EDGE('',*,*,#13999,.T.);
#18265=ORIENTED_EDGE('',*,*,#14004,.F.);
#18266=ORIENTED_EDGE('',*,*,#14005,.F.);
#18267=ORIENTED_EDGE('',*,*,#14006,.T.);
#18268=ORIENTED_EDGE('',*,*,#14002,.T.);
#18269=ORIENTED_EDGE('',*,*,#14007,.F.);
#18270=ORIENTED_EDGE('',*,*,#14008,.F.);
#18271=ORIENTED_EDGE('',*,*,#14009,.T.);
#18272=ORIENTED_EDGE('',*,*,#14005,.T.);
#18273=ORIENTED_EDGE('',*,*,#14010,.F.);
#18274=ORIENTED_EDGE('',*,*,#14011,.F.);
#18275=ORIENTED_EDGE('',*,*,#14012,.T.);
#18276=ORIENTED_EDGE('',*,*,#14008,.T.);
#18277=ORIENTED_EDGE('',*,*,#14013,.F.);
#18278=ORIENTED_EDGE('',*,*,#14014,.F.);
#18279=ORIENTED_EDGE('',*,*,#14015,.T.);
#18280=ORIENTED_EDGE('',*,*,#14011,.T.);
#18281=ORIENTED_EDGE('',*,*,#14016,.F.);
#18282=ORIENTED_EDGE('',*,*,#14017,.F.);
#18283=ORIENTED_EDGE('',*,*,#14018,.T.);
#18284=ORIENTED_EDGE('',*,*,#14014,.T.);
#18285=ORIENTED_EDGE('',*,*,#14019,.F.);
#18286=ORIENTED_EDGE('',*,*,#14020,.F.);
#18287=ORIENTED_EDGE('',*,*,#14021,.T.);
#18288=ORIENTED_EDGE('',*,*,#14017,.T.);
#18289=ORIENTED_EDGE('',*,*,#14022,.F.);
#18290=ORIENTED_EDGE('',*,*,#14023,.F.);
#18291=ORIENTED_EDGE('',*,*,#14024,.T.);
#18292=ORIENTED_EDGE('',*,*,#14020,.T.);
#18293=ORIENTED_EDGE('',*,*,#14025,.F.);
#18294=ORIENTED_EDGE('',*,*,#14026,.F.);
#18295=ORIENTED_EDGE('',*,*,#14027,.T.);
#18296=ORIENTED_EDGE('',*,*,#14023,.T.);
#18297=ORIENTED_EDGE('',*,*,#14028,.F.);
#18298=ORIENTED_EDGE('',*,*,#14029,.F.);
#18299=ORIENTED_EDGE('',*,*,#14030,.T.);
#18300=ORIENTED_EDGE('',*,*,#14026,.T.);
#18301=ORIENTED_EDGE('',*,*,#14031,.F.);
#18302=ORIENTED_EDGE('',*,*,#13997,.T.);
#18303=ORIENTED_EDGE('',*,*,#13994,.T.);
#18304=ORIENTED_EDGE('',*,*,#14032,.T.);
#18305=ORIENTED_EDGE('',*,*,#14033,.F.);
#18306=ORIENTED_EDGE('',*,*,#14034,.F.);
#18307=ORIENTED_EDGE('',*,*,#14035,.T.);
#18308=ORIENTED_EDGE('',*,*,#14035,.F.);
#18309=ORIENTED_EDGE('',*,*,#14036,.F.);
#18310=ORIENTED_EDGE('',*,*,#13991,.F.);
#18311=ORIENTED_EDGE('',*,*,#13988,.F.);
#18312=ORIENTED_EDGE('',*,*,#13985,.F.);
#18313=ORIENTED_EDGE('',*,*,#13982,.F.);
#18314=ORIENTED_EDGE('',*,*,#13979,.F.);
#18315=ORIENTED_EDGE('',*,*,#13976,.F.);
#18316=ORIENTED_EDGE('',*,*,#13973,.F.);
#18317=ORIENTED_EDGE('',*,*,#13970,.F.);
#18318=ORIENTED_EDGE('',*,*,#13967,.F.);
#18319=ORIENTED_EDGE('',*,*,#13964,.F.);
#18320=ORIENTED_EDGE('',*,*,#13961,.F.);
#18321=ORIENTED_EDGE('',*,*,#13958,.F.);
#18322=ORIENTED_EDGE('',*,*,#13955,.F.);
#18323=ORIENTED_EDGE('',*,*,#14037,.F.);
#18324=ORIENTED_EDGE('',*,*,#14038,.T.);
#18325=ORIENTED_EDGE('',*,*,#14031,.T.);
#18326=ORIENTED_EDGE('',*,*,#14028,.T.);
#18327=ORIENTED_EDGE('',*,*,#14025,.T.);
#18328=ORIENTED_EDGE('',*,*,#14022,.T.);
#18329=ORIENTED_EDGE('',*,*,#14019,.T.);
#18330=ORIENTED_EDGE('',*,*,#14016,.T.);
#18331=ORIENTED_EDGE('',*,*,#14013,.T.);
#18332=ORIENTED_EDGE('',*,*,#14010,.T.);
#18333=ORIENTED_EDGE('',*,*,#14007,.T.);
#18334=ORIENTED_EDGE('',*,*,#14004,.T.);
#18335=ORIENTED_EDGE('',*,*,#14001,.T.);
#18336=ORIENTED_EDGE('',*,*,#13998,.T.);
#18337=ORIENTED_EDGE('',*,*,#14039,.T.);
#18338=ORIENTED_EDGE('',*,*,#14040,.T.);
#18339=ORIENTED_EDGE('',*,*,#14041,.T.);
#18340=ORIENTED_EDGE('',*,*,#14042,.T.);
#18341=ORIENTED_EDGE('',*,*,#14037,.T.);
#18342=ORIENTED_EDGE('',*,*,#14029,.T.);
#18343=ORIENTED_EDGE('',*,*,#14038,.F.);
#18344=ORIENTED_EDGE('',*,*,#14042,.F.);
#18345=ORIENTED_EDGE('',*,*,#14043,.T.);
#18346=ORIENTED_EDGE('',*,*,#14032,.F.);
#18347=ORIENTED_EDGE('',*,*,#13993,.F.);
#18348=ORIENTED_EDGE('',*,*,#13996,.F.);
#18349=ORIENTED_EDGE('',*,*,#14000,.F.);
#18350=ORIENTED_EDGE('',*,*,#14003,.F.);
#18351=ORIENTED_EDGE('',*,*,#14006,.F.);
#18352=ORIENTED_EDGE('',*,*,#14009,.F.);
#18353=ORIENTED_EDGE('',*,*,#14012,.F.);
#18354=ORIENTED_EDGE('',*,*,#14015,.F.);
#18355=ORIENTED_EDGE('',*,*,#14018,.F.);
#18356=ORIENTED_EDGE('',*,*,#14021,.F.);
#18357=ORIENTED_EDGE('',*,*,#14024,.F.);
#18358=ORIENTED_EDGE('',*,*,#14027,.F.);
#18359=ORIENTED_EDGE('',*,*,#14030,.F.);
#18360=ORIENTED_EDGE('',*,*,#14043,.F.);
#18361=ORIENTED_EDGE('',*,*,#14041,.F.);
#18362=ORIENTED_EDGE('',*,*,#13953,.F.);
#18363=ORIENTED_EDGE('',*,*,#13957,.F.);
#18364=ORIENTED_EDGE('',*,*,#13960,.F.);
#18365=ORIENTED_EDGE('',*,*,#13963,.F.);
#18366=ORIENTED_EDGE('',*,*,#13966,.F.);
#18367=ORIENTED_EDGE('',*,*,#13969,.F.);
#18368=ORIENTED_EDGE('',*,*,#13972,.F.);
#18369=ORIENTED_EDGE('',*,*,#13975,.F.);
#18370=ORIENTED_EDGE('',*,*,#13978,.F.);
#18371=ORIENTED_EDGE('',*,*,#13981,.F.);
#18372=ORIENTED_EDGE('',*,*,#13984,.F.);
#18373=ORIENTED_EDGE('',*,*,#13987,.F.);
#18374=ORIENTED_EDGE('',*,*,#13990,.F.);
#18375=ORIENTED_EDGE('',*,*,#14044,.F.);
#18376=ORIENTED_EDGE('',*,*,#13989,.T.);
#18377=ORIENTED_EDGE('',*,*,#14036,.T.);
#18378=ORIENTED_EDGE('',*,*,#14045,.F.);
#18379=ORIENTED_EDGE('',*,*,#14044,.T.);
#18380=ORIENTED_EDGE('',*,*,#14046,.F.);
#18381=ORIENTED_EDGE('',*,*,#14047,.F.);
#18382=ORIENTED_EDGE('',*,*,#14048,.T.);
#18383=ORIENTED_EDGE('',*,*,#14046,.T.);
#18384=ORIENTED_EDGE('',*,*,#14048,.F.);
#18385=ORIENTED_EDGE('',*,*,#14049,.F.);
#18386=ORIENTED_EDGE('',*,*,#14050,.T.);
#18387=ORIENTED_EDGE('',*,*,#14047,.T.);
#18388=ORIENTED_EDGE('',*,*,#14050,.F.);
#18389=ORIENTED_EDGE('',*,*,#14049,.T.);
#18390=ORIENTED_EDGE('',*,*,#14051,.F.);
#18391=ORIENTED_EDGE('',*,*,#14039,.F.);
#18392=ORIENTED_EDGE('',*,*,#13954,.F.);
#18393=ORIENTED_EDGE('',*,*,#14040,.F.);
#18394=ORIENTED_EDGE('',*,*,#14052,.T.);
#18395=ORIENTED_EDGE('',*,*,#14051,.T.);
#18396=ORIENTED_EDGE('',*,*,#14052,.F.);
#18397=ORIENTED_EDGE('',*,*,#14053,.F.);
#18398=ORIENTED_EDGE('',*,*,#14054,.T.);
#18399=ORIENTED_EDGE('',*,*,#14033,.T.);
#18400=ORIENTED_EDGE('',*,*,#14045,.T.);
#18401=ORIENTED_EDGE('',*,*,#14034,.T.);
#18402=ORIENTED_EDGE('',*,*,#14054,.F.);
#18403=ORIENTED_EDGE('',*,*,#14053,.T.);
#25296=CONICAL_SURFACE('',#27273,1.85,0.785398163397447);
#25297=CONICAL_SURFACE('',#27279,1.225,0.785398163397477);
#25298=CONICAL_SURFACE('',#27280,1.125,0.785398163397453);
#25507=ADVANCED_FACE('',(#2694),#558,.T.);
#25508=ADVANCED_FACE('',(#2695),#559,.T.);
#25509=ADVANCED_FACE('',(#2696),#560,.T.);
#25510=ADVANCED_FACE('',(#2697),#561,.T.);
#25511=ADVANCED_FACE('',(#2698),#562,.T.);
#25512=ADVANCED_FACE('',(#2699),#563,.T.);
#25513=ADVANCED_FACE('',(#2700),#564,.T.);
#25514=ADVANCED_FACE('',(#2701),#565,.T.);
#25515=ADVANCED_FACE('',(#2702),#566,.T.);
#25516=ADVANCED_FACE('',(#2703),#567,.T.);
#25517=ADVANCED_FACE('',(#2704),#568,.T.);
#25518=ADVANCED_FACE('',(#2705),#569,.T.);
#25519=ADVANCED_FACE('',(#2706),#570,.T.);
#25520=ADVANCED_FACE('',(#2707),#571,.T.);
#25521=ADVANCED_FACE('',(#2708),#572,.T.);
#25522=ADVANCED_FACE('',(#2709),#573,.T.);
#25523=ADVANCED_FACE('',(#2710),#574,.T.);
#25524=ADVANCED_FACE('',(#2711),#575,.T.);
#25525=ADVANCED_FACE('',(#2712),#576,.T.);
#25526=ADVANCED_FACE('',(#2713),#577,.T.);
#25527=ADVANCED_FACE('',(#2714),#578,.T.);
#25528=ADVANCED_FACE('',(#2715),#579,.T.);
#25529=ADVANCED_FACE('',(#2716),#580,.T.);
#25530=ADVANCED_FACE('',(#2717),#581,.T.);
#25531=ADVANCED_FACE('',(#2718),#582,.T.);
#25532=ADVANCED_FACE('',(#2719),#583,.T.);
#25533=ADVANCED_FACE('',(#2720),#1722,.F.);
#25534=ADVANCED_FACE('',(#2721),#270,.F.);
#25535=ADVANCED_FACE('',(#2722),#1723,.T.);
#25536=ADVANCED_FACE('',(#2723),#584,.T.);
#25537=ADVANCED_FACE('',(#2724),#271,.F.);
#25538=ADVANCED_FACE('',(#2725),#585,.T.);
#25539=ADVANCED_FACE('',(#2726),#1724,.T.);
#25540=ADVANCED_FACE('',(#2727),#25296,.T.);
#25541=ADVANCED_FACE('',(#2728),#586,.T.);
#25542=ADVANCED_FACE('',(#2729,#849),#1725,.T.);
#25543=ADVANCED_FACE('',(#2730),#25297,.T.);
#25544=ADVANCED_FACE('',(#2731),#25298,.T.);
#25545=ADVANCED_FACE('',(#2732),#1726,.T.);
#26873=CLOSED_SHELL('',(#25507,#25508,#25509,#25510,#25511,#25512,#25513,
#25514,#25515,#25516,#25517,#25518,#25519,#25520,#25521,#25522,#25523,#25524,
#25525,#25526,#25527,#25528,#25529,#25530,#25531,#25532,#25533,#25534,#25535,
#25536,#25537,#25538,#25539,#25540,#25541,#25542,#25543,#25544,#25545));
#27231=AXIS2_PLACEMENT_3D('',#40322,#29495,#29496);
#27232=AXIS2_PLACEMENT_3D('',#40323,#29497,#29498);
#27233=AXIS2_PLACEMENT_3D('',#40345,#29500,#29501);
#27234=AXIS2_PLACEMENT_3D('',#40356,#29502,#29503);
#27235=AXIS2_PLACEMENT_3D('',#40440,#29505,#29506);
#27236=AXIS2_PLACEMENT_3D('',#40530,#29508,#29509);
#27237=AXIS2_PLACEMENT_3D('',#40620,#29511,#29512);
#27238=AXIS2_PLACEMENT_3D('',#40704,#29514,#29515);
#27239=AXIS2_PLACEMENT_3D('',#40794,#29517,#29518);
#27240=AXIS2_PLACEMENT_3D('',#40878,#29520,#29521);
#27241=AXIS2_PLACEMENT_3D('',#40968,#29523,#29524);
#27242=AXIS2_PLACEMENT_3D('',#41058,#29526,#29527);
#27243=AXIS2_PLACEMENT_3D('',#41142,#29529,#29530);
#27244=AXIS2_PLACEMENT_3D('',#41232,#29532,#29533);
#27245=AXIS2_PLACEMENT_3D('',#41322,#29535,#29536);
#27246=AXIS2_PLACEMENT_3D('',#41406,#29538,#29539);
#27247=AXIS2_PLACEMENT_3D('',#41415,#29541,#29542);
#27248=AXIS2_PLACEMENT_3D('',#41416,#29543,#29544);
#27249=AXIS2_PLACEMENT_3D('',#41437,#29546,#29547);
#27250=AXIS2_PLACEMENT_3D('',#41452,#29548,#29549);
#27251=AXIS2_PLACEMENT_3D('',#41489,#29551,#29552);
#27252=AXIS2_PLACEMENT_3D('',#41527,#29554,#29555);
#27253=AXIS2_PLACEMENT_3D('',#41564,#29557,#29558);
#27254=AXIS2_PLACEMENT_3D('',#41601,#29560,#29561);
#27255=AXIS2_PLACEMENT_3D('',#41639,#29563,#29564);
#27256=AXIS2_PLACEMENT_3D('',#41676,#29566,#29567);
#27257=AXIS2_PLACEMENT_3D('',#41713,#29569,#29570);
#27258=AXIS2_PLACEMENT_3D('',#41750,#29572,#29573);
#27259=AXIS2_PLACEMENT_3D('',#41787,#29575,#29576);
#27260=AXIS2_PLACEMENT_3D('',#41825,#29578,#29579);
#27261=AXIS2_PLACEMENT_3D('',#41862,#29581,#29582);
#27262=AXIS2_PLACEMENT_3D('',#41944,#29583,#29584);
#27263=AXIS2_PLACEMENT_3D('',#41946,#29585,#29586);
#27264=AXIS2_PLACEMENT_3D('',#42813,#29587,#29588);
#27265=AXIS2_PLACEMENT_3D('',#42815,#29589,#29590);
#27266=AXIS2_PLACEMENT_3D('',#42816,#29591,#29592);
#27267=AXIS2_PLACEMENT_3D('',#42900,#29593,#29594);
#27268=AXIS2_PLACEMENT_3D('',#42901,#29595,#29596);
#27269=AXIS2_PLACEMENT_3D('',#43598,#29597,#29598);
#27270=AXIS2_PLACEMENT_3D('',#43599,#29599,#29600);
#27271=AXIS2_PLACEMENT_3D('',#43600,#29601,#29602);
#27272=AXIS2_PLACEMENT_3D('',#43602,#29603,#29604);
#27273=AXIS2_PLACEMENT_3D('',#43603,#29605,#29606);
#27274=AXIS2_PLACEMENT_3D('',#43605,#29607,#29608);
#27275=AXIS2_PLACEMENT_3D('',#43607,#29610,#29611);
#27276=AXIS2_PLACEMENT_3D('',#43609,#29612,#29613);
#27277=AXIS2_PLACEMENT_3D('',#43611,#29615,#29616);
#27278=AXIS2_PLACEMENT_3D('',#43613,#29617,#29618);
#27279=AXIS2_PLACEMENT_3D('',#43614,#29619,#29620);
#27280=AXIS2_PLACEMENT_3D('',#43616,#29622,#29623);
#27281=AXIS2_PLACEMENT_3D('',#43618,#29624,#29625);
#27282=AXIS2_PLACEMENT_3D('',#43620,#29627,#29628);
#29495=DIRECTION('axis',(0.,0.,1.));
#29496=DIRECTION('refdir',(1.,0.,0.));
#29497=DIRECTION('center_axis',(0.,0.,1.));
#29498=DIRECTION('ref_axis',(1.,0.,0.));
#29499=DIRECTION('',(0.,0.,-1.));
#29500=DIRECTION('center_axis',(0.,0.,-1.));
#29501=DIRECTION('ref_axis',(1.,0.,0.));
#29502=DIRECTION('center_axis',(0.,0.,1.));
#29503=DIRECTION('ref_axis',(1.,0.,0.));
#29504=DIRECTION('',(0.,0.,-1.));
#29505=DIRECTION('center_axis',(0.,0.,1.));
#29506=DIRECTION('ref_axis',(1.,0.,0.));
#29507=DIRECTION('',(0.,0.,-1.));
#29508=DIRECTION('center_axis',(0.,0.,1.));
#29509=DIRECTION('ref_axis',(1.,0.,0.));
#29510=DIRECTION('',(0.,0.,-1.));
#29511=DIRECTION('center_axis',(0.,0.,1.));
#29512=DIRECTION('ref_axis',(1.,0.,0.));
#29513=DIRECTION('',(0.,0.,-1.));
#29514=DIRECTION('center_axis',(0.,0.,1.));
#29515=DIRECTION('ref_axis',(1.,0.,0.));
#29516=DIRECTION('',(0.,0.,-1.));
#29517=DIRECTION('center_axis',(0.,0.,1.));
#29518=DIRECTION('ref_axis',(1.,0.,0.));
#29519=DIRECTION('',(0.,0.,-1.));
#29520=DIRECTION('center_axis',(0.,0.,1.));
#29521=DIRECTION('ref_axis',(1.,0.,0.));
#29522=DIRECTION('',(0.,0.,-1.));
#29523=DIRECTION('center_axis',(0.,0.,1.));
#29524=DIRECTION('ref_axis',(1.,0.,0.));
#29525=DIRECTION('',(0.,0.,-1.));
#29526=DIRECTION('center_axis',(0.,0.,1.));
#29527=DIRECTION('ref_axis',(1.,0.,0.));
#29528=DIRECTION('',(0.,0.,-1.));
#29529=DIRECTION('center_axis',(0.,0.,1.));
#29530=DIRECTION('ref_axis',(1.,0.,0.));
#29531=DIRECTION('',(0.,0.,-1.));
#29532=DIRECTION('center_axis',(0.,0.,1.));
#29533=DIRECTION('ref_axis',(1.,0.,0.));
#29534=DIRECTION('',(0.,0.,-1.));
#29535=DIRECTION('center_axis',(0.,0.,1.));
#29536=DIRECTION('ref_axis',(1.,0.,0.));
#29537=DIRECTION('',(0.,0.,-1.));
#29538=DIRECTION('center_axis',(0.,0.,1.));
#29539=DIRECTION('ref_axis',(1.,7.08873565758722E-14,0.));
#29540=DIRECTION('',(0.,0.,1.));
#29541=DIRECTION('center_axis',(0.,0.,1.));
#29542=DIRECTION('ref_axis',(1.,7.08873565758722E-14,0.));
#29543=DIRECTION('center_axis',(0.,0.,1.));
#29544=DIRECTION('ref_axis',(1.,7.08873565758722E-14,0.));
#29545=DIRECTION('',(0.,0.,1.));
#29546=DIRECTION('center_axis',(0.,0.,1.));
#29547=DIRECTION('ref_axis',(1.,7.08873565758722E-14,0.));
#29548=DIRECTION('center_axis',(0.,0.,1.));
#29549=DIRECTION('ref_axis',(1.,7.08873565758722E-14,0.));
#29550=DIRECTION('',(0.,0.,1.));
#29551=DIRECTION('center_axis',(0.,0.,1.));
#29552=DIRECTION('ref_axis',(1.,7.08873565758722E-14,0.));
#29553=DIRECTION('',(0.,0.,1.));
#29554=DIRECTION('center_axis',(0.,0.,1.));
#29555=DIRECTION('ref_axis',(1.,7.08873565758722E-14,0.));
#29556=DIRECTION('',(0.,0.,1.));
#29557=DIRECTION('center_axis',(0.,0.,1.));
#29558=DIRECTION('ref_axis',(1.,7.08873565758722E-14,0.));
#29559=DIRECTION('',(0.,0.,1.));
#29560=DIRECTION('center_axis',(0.,0.,1.));
#29561=DIRECTION('ref_axis',(1.,7.08873565758722E-14,0.));
#29562=DIRECTION('',(0.,0.,1.));
#29563=DIRECTION('center_axis',(0.,0.,1.));
#29564=DIRECTION('ref_axis',(1.,7.08873565758722E-14,0.));
#29565=DIRECTION('',(0.,0.,1.));
#29566=DIRECTION('center_axis',(0.,0.,1.));
#29567=DIRECTION('ref_axis',(1.,7.08873565758722E-14,0.));
#29568=DIRECTION('',(0.,0.,1.));
#29569=DIRECTION('center_axis',(0.,0.,1.));
#29570=DIRECTION('ref_axis',(1.,7.08873565758722E-14,0.));
#29571=DIRECTION('',(0.,0.,1.));
#29572=DIRECTION('center_axis',(0.,0.,1.));
#29573=DIRECTION('ref_axis',(1.,7.08873565758722E-14,0.));
#29574=DIRECTION('',(0.,0.,1.));
#29575=DIRECTION('center_axis',(0.,0.,1.));
#29576=DIRECTION('ref_axis',(1.,7.08873565758722E-14,0.));
#29577=DIRECTION('',(0.,0.,1.));
#29578=DIRECTION('center_axis',(0.,0.,1.));
#29579=DIRECTION('ref_axis',(1.,7.08873565758722E-14,0.));
#29580=DIRECTION('',(0.,0.,1.));
#29581=DIRECTION('center_axis',(0.,0.,1.));
#29582=DIRECTION('ref_axis',(1.,0.,0.));
#29583=DIRECTION('center_axis',(0.,0.,-1.));
#29584=DIRECTION('ref_axis',(1.,0.,0.));
#29585=DIRECTION('center_axis',(0.,0.,-1.));
#29586=DIRECTION('ref_axis',(1.,0.,0.));
#29587=DIRECTION('center_axis',(0.,0.,1.));
#29588=DIRECTION('ref_axis',(1.,0.,0.));
#29589=DIRECTION('center_axis',(0.,0.,-1.));
#29590=DIRECTION('ref_axis',(1.,0.,0.));
#29591=DIRECTION('center_axis',(0.,0.,-1.));
#29592=DIRECTION('ref_axis',(1.,0.,0.));
#29593=DIRECTION('center_axis',(0.,0.,-1.));
#29594=DIRECTION('ref_axis',(1.,7.08873565758722E-14,0.));
#29595=DIRECTION('center_axis',(0.,0.,1.));
#29596=DIRECTION('ref_axis',(0.888987612330369,0.457931244973685,0.));
#29597=DIRECTION('center_axis',(0.,0.,1.));
#29598=DIRECTION('ref_axis',(1.,0.,0.));
#29599=DIRECTION('center_axis',(0.,0.,-1.));
#29600=DIRECTION('ref_axis',(1.,0.,0.));
#29601=DIRECTION('center_axis',(0.,0.,-1.));
#29602=DIRECTION('ref_axis',(-1.,0.,0.));
#29603=DIRECTION('center_axis',(0.,0.,1.));
#29604=DIRECTION('ref_axis',(1.,0.,0.));
#29605=DIRECTION('center_axis',(0.,0.,1.));
#29606=DIRECTION('ref_axis',(1.,0.,0.));
#29607=DIRECTION('center_axis',(0.,0.,1.));
#29608=DIRECTION('ref_axis',(1.,0.,0.));
#29609=DIRECTION('',(0.707106781186547,8.65956056235492E-17,-0.707106781186548));
#29610=DIRECTION('center_axis',(0.,0.,1.));
#29611=DIRECTION('ref_axis',(1.,0.,0.));
#29612=DIRECTION('center_axis',(0.,0.,1.));
#29613=DIRECTION('ref_axis',(1.,0.,0.));
#29614=DIRECTION('',(0.,0.,-1.));
#29615=DIRECTION('center_axis',(0.,0.,1.));
#29616=DIRECTION('ref_axis',(1.,0.,0.));
#29617=DIRECTION('center_axis',(0.,0.,1.));
#29618=DIRECTION('ref_axis',(1.,0.,0.));
#29619=DIRECTION('center_axis',(0.,0.,-1.));
#29620=DIRECTION('ref_axis',(1.,0.,0.));
#29621=DIRECTION('',(-0.707106781186568,-8.65956056235518E-17,-0.707106781186527));
#29622=DIRECTION('center_axis',(0.,0.,-1.));
#29623=DIRECTION('ref_axis',(1.,0.,0.));
#29624=DIRECTION('center_axis',(0.,0.,1.));
#29625=DIRECTION('ref_axis',(1.,0.,0.));
#29626=DIRECTION('',(-0.707106781186551,-8.65956056235497E-17,-0.707106781186544));
#29627=DIRECTION('center_axis',(0.,0.,1.));
#29628=DIRECTION('ref_axis',(1.,0.,0.));
#40322=CARTESIAN_POINT('',(0.,0.,0.));
#40323=CARTESIAN_POINT('Origin',(0.,0.,57.95));
#40324=CARTESIAN_POINT('',(-1.18823416249667,3.04042717342579E-5,56.1580381236952));
#40325=CARTESIAN_POINT('',(-1.1882111814849,2.07922408733904E-5,56.1155118763048));
#40326=CARTESIAN_POINT('',(-1.188225,-1.45515594291686E-16,57.95));
#40327=CARTESIAN_POINT('',(0.511859986942129,1.07234629461565,56.061775));
#40328=CARTESIAN_POINT('Ctrl Pts',(-1.18823416249667,3.04042717342579E-5,
56.1580381236952));
#40329=CARTESIAN_POINT('Ctrl Pts',(-1.18827861610379,0.0433316730233904,
56.1562980870114));
#40330=CARTESIAN_POINT('Ctrl Pts',(-1.18595724154989,0.0866281961938818,
56.1545580503277));
#40331=CARTESIAN_POINT('Ctrl Pts',(-1.18123364237345,0.129661025825523,
56.1528180136439));
#40332=CARTESIAN_POINT('Ctrl Pts',(-1.15971967143524,0.325657132078954,
56.1448928918782));
#40333=CARTESIAN_POINT('Ctrl Pts',(-1.08837365745739,0.516183147128608,
56.1369677701125));
#40334=CARTESIAN_POINT('Ctrl Pts',(-0.975859421229326,0.678102705033355,
56.1290426483468));
#40335=CARTESIAN_POINT('Ctrl Pts',(-0.863345185001266,0.840022262938101,
56.121117526581));
#40336=CARTESIAN_POINT('Ctrl Pts',(-0.709662726523,0.973335363697939,56.1131924048153));
#40337=CARTESIAN_POINT('Ctrl Pts',(-0.5334751176618,1.06185197282687,56.1052672830496));
#40338=CARTESIAN_POINT('Ctrl Pts',(-0.357287508800601,1.15036858195579,
56.0973421612839));
#40339=CARTESIAN_POINT('Ctrl Pts',(-0.158594749556469,1.19408869945381,
56.0894170395182));
#40340=CARTESIAN_POINT('Ctrl Pts',(0.0384754792288307,1.18770519465287,
56.0814919177524));
#40341=CARTESIAN_POINT('Ctrl Pts',(0.201905880564523,1.18241135215836,56.074919611835));
#40342=CARTESIAN_POINT('Ctrl Pts',(0.364220404424889,1.14265929456453,56.0683473059175));
#40343=CARTESIAN_POINT('Ctrl Pts',(0.511881162716727,1.07235883428017,56.061775));
#40344=CARTESIAN_POINT('',(-0.511838811167444,1.07233375495118,56.061775));
#40345=CARTESIAN_POINT('Origin',(0.,0.,56.061775));
#40346=CARTESIAN_POINT('Ctrl Pts',(-0.511838811167444,1.07233375495118,
56.061775));
#40347=CARTESIAN_POINT('Ctrl Pts',(-0.689828373128891,0.987377028210158,
56.0697001217657));
#40348=CARTESIAN_POINT('Ctrl Pts',(-0.846158719658857,0.857268871760102,
56.0776252435314));
#40349=CARTESIAN_POINT('Ctrl Pts',(-0.961924008494834,0.697685904838996,
56.0855503652972));
#40350=CARTESIAN_POINT('Ctrl Pts',(-1.07768929733081,0.538102937917886,
56.0934754870629));
#40351=CARTESIAN_POINT('Ctrl Pts',(-1.1528895284728,0.349045160525724,56.1014006088286));
#40352=CARTESIAN_POINT('Ctrl Pts',(-1.17836884940845,0.153522240919442,
56.1093257305943));
#40353=CARTESIAN_POINT('Ctrl Pts',(-1.18499834973128,0.102648857679571,
56.1113877791645));
#40354=CARTESIAN_POINT('Ctrl Pts',(-1.18826176594027,0.0513377871083471,
56.1134498277346));
#40355=CARTESIAN_POINT('Ctrl Pts',(-1.1882111814849,2.07922408733904E-5,
56.1155118763048));
#40356=CARTESIAN_POINT('Origin',(0.,0.,57.95));
#40357=CARTESIAN_POINT('',(-1.18826932065667,-2.69461188108222E-5,56.4580381236952));
#40358=CARTESIAN_POINT('',(-1.18829206995915,-2.22507172762053E-5,56.4155118763048));
#40359=CARTESIAN_POINT('',(-1.188225,-1.45515594291686E-16,57.95));
#40360=CARTESIAN_POINT('Ctrl Pts',(-1.18826932065667,-2.69461188108222E-5,
56.4580381236952));
#40361=CARTESIAN_POINT('Ctrl Pts',(-1.18810768463847,0.165161660669492,
56.4513995482));
#40362=CARTESIAN_POINT('Ctrl Pts',(-1.15335574970162,0.330416144443476,
56.4447609727049));
#40363=CARTESIAN_POINT('Ctrl Pts',(-1.0864436295599,0.481419953396779,56.4381223972098));
#40364=CARTESIAN_POINT('Ctrl Pts',(-1.00656403790443,0.661688080786279,
56.430197275444));
#40365=CARTESIAN_POINT('Ctrl Pts',(-0.880851198609791,0.821646788192008,
56.4222721536783));
#40366=CARTESIAN_POINT('Ctrl Pts',(-0.724571239081175,0.941871249812796,
56.4143470319126));
#40367=CARTESIAN_POINT('Ctrl Pts',(-0.568291279552556,1.06209571143359,
56.4064219101469));
#40368=CARTESIAN_POINT('Ctrl Pts',(-0.381444199789957,1.14258592726943,
56.3984967883812));
#40369=CARTESIAN_POINT('Ctrl Pts',(-0.18672005555549,1.17356744699151,56.3905716666154));
#40370=CARTESIAN_POINT('Ctrl Pts',(0.00800408867897459,1.20454896671359,
56.3826465448497));
#40371=CARTESIAN_POINT('Ctrl Pts',(0.210605297385308,1.1860217903219,56.374721423084));
#40372=CARTESIAN_POINT('Ctrl Pts',(0.396480388623666,1.12023579351038,56.3667963013183));
#40373=CARTESIAN_POINT('Ctrl Pts',(0.582355479862024,1.05444979669886,56.3588711795526));
#40374=CARTESIAN_POINT('Ctrl Pts',(0.751504453632407,0.941404979467515,
56.3509460577869));
#40375=CARTESIAN_POINT('Ctrl Pts',(0.883386450102643,0.794829108512784,
56.3430209360211));
#40376=CARTESIAN_POINT('Ctrl Pts',(1.01526844657288,0.648253237558053,56.3350958142554));
#40377=CARTESIAN_POINT('Ctrl Pts',(1.10988346574297,0.468146312879939,56.3271706924897));
#40378=CARTESIAN_POINT('Ctrl Pts',(1.15574179108387,0.276379890303732,56.319245570724));
#40379=CARTESIAN_POINT('Ctrl Pts',(1.20160011642478,0.0846134677275266,
56.3113204489583));
#40380=CARTESIAN_POINT('Ctrl Pts',(1.1987017479365,-0.118812452746773,56.3033953271926));
#40381=CARTESIAN_POINT('Ctrl Pts',(1.14739865246892,-0.30919454104491,56.2954702054269));
#40382=CARTESIAN_POINT('Ctrl Pts',(1.09609555700134,-0.499576629343047,
56.2875450836611));
#40383=CARTESIAN_POINT('Ctrl Pts',(0.996387734554462,-0.676914885465023,
56.2796199618954));
#40384=CARTESIAN_POINT('Ctrl Pts',(0.860383356175942,-0.81967396751617,
56.2716948401297));
#40385=CARTESIAN_POINT('Ctrl Pts',(0.72437897779742,-0.962433049567319,
56.263769718364));
#40386=CARTESIAN_POINT('Ctrl Pts',(0.552078043487259,-1.07061295754764,
56.2558445965983));
#40387=CARTESIAN_POINT('Ctrl Pts',(0.364404171862087,-1.13107671147003,
56.2479194748325));
#40388=CARTESIAN_POINT('Ctrl Pts',(0.176730300236916,-1.19154046539241,
56.2399943530668));
#40389=CARTESIAN_POINT('Ctrl Pts',(-0.0263165087032649,-1.20428806525687,
56.2320692313011));
#40390=CARTESIAN_POINT('Ctrl Pts',(-0.220078951989418,-1.1677714664526,
56.2241441095354));
#40391=CARTESIAN_POINT('Ctrl Pts',(-0.41384139527557,-1.13125486764833,
56.2162189877697));
#40392=CARTESIAN_POINT('Ctrl Pts',(-0.598319472907694,-1.04547407017534,
56.2082938660039));
#40393=CARTESIAN_POINT('Ctrl Pts',(-0.751110831485251,-0.920846038545505,
56.2003687442382));
#40394=CARTESIAN_POINT('Ctrl Pts',(-0.903902190062808,-0.796218006915672,
56.1924436224725));
#40395=CARTESIAN_POINT('Ctrl Pts',(-1.0250068295858,-0.632742741128994,
56.1845185007068));
#40396=CARTESIAN_POINT('Ctrl Pts',(-1.09971818539801,-0.450272009507053,
56.1765933789411));
#40397=CARTESIAN_POINT('Ctrl Pts',(-1.15802594469153,-0.307864481469854,
56.1704082938591));
#40398=CARTESIAN_POINT('Ctrl Pts',(-1.18807614896463,-0.153887058438266,
56.1642232087771));
#40399=CARTESIAN_POINT('Ctrl Pts',(-1.18823416249667,3.04042717342579E-5,
56.1580381236952));
#40400=CARTESIAN_POINT('Ctrl Pts',(-1.1882111814849,2.07922408733904E-5,
56.1155118763048));
#40401=CARTESIAN_POINT('Ctrl Pts',(-1.18806735346424,-0.145890075929576,
56.1213749495004));
#40402=CARTESIAN_POINT('Ctrl Pts',(-1.16113150647432,-0.291848839038371,
56.1272380226959));
#40403=CARTESIAN_POINT('Ctrl Pts',(-1.10860087444441,-0.427930629202327,
56.1331010958914));
#40404=CARTESIAN_POINT('Ctrl Pts',(-1.03759516781542,-0.611872517897413,
56.1410262176572));
#40405=CARTESIAN_POINT('Ctrl Pts',(-0.919825343828156,-0.777768233467184,
56.1489513394229));
#40406=CARTESIAN_POINT('Ctrl Pts',(-0.769587398025842,-0.905462855000406,
56.1568764611886));
#40407=CARTESIAN_POINT('Ctrl Pts',(-0.619349452223529,-1.03315747653363,
56.1648015829543));
#40408=CARTESIAN_POINT('Ctrl Pts',(-0.43664338460617,-1.1226510040303,56.17272670472));
#40409=CARTESIAN_POINT('Ctrl Pts',(-0.243659060499568,-1.16307964514265,
56.1806518264858));
#40410=CARTESIAN_POINT('Ctrl Pts',(-0.0506747363929658,-1.203508286255,
56.1885769482515));
#40411=CARTESIAN_POINT('Ctrl Pts',(0.15258784420288,-1.19487204098302,56.1965020700172));
#40412=CARTESIAN_POINT('Ctrl Pts',(0.341446405860296,-1.13821776082292,
56.2044271917829));
#40413=CARTESIAN_POINT('Ctrl Pts',(0.530304967517711,-1.08156348066281,
56.2123523135486));
#40414=CARTESIAN_POINT('Ctrl Pts',(0.704759510236697,-0.976891165614581,
56.2202774353144));
#40415=CARTESIAN_POINT('Ctrl Pts',(0.843624313143388,-0.836912727100357,
56.2282025570801));
#40416=CARTESIAN_POINT('Ctrl Pts',(0.982489116050078,-0.696934288586134,
56.2361276788458));
#40417=CARTESIAN_POINT('Ctrl Pts',(1.08576417914447,-0.521649726605918,
56.2440528006115));
#40418=CARTESIAN_POINT('Ctrl Pts',(1.14090840415554,-0.332344578155793,
56.2519779223772));
#40419=CARTESIAN_POINT('Ctrl Pts',(1.1960526291666,-0.143039429705667,56.2599030441429));
#40420=CARTESIAN_POINT('Ctrl Pts',(1.20306601609434,0.0602863052143686,
56.2678281659087));
#40421=CARTESIAN_POINT('Ctrl Pts',(1.16109676099022,0.252941272364512,56.2757532876744));
#40422=CARTESIAN_POINT('Ctrl Pts',(1.1191275058861,0.445596239514657,56.2836784094401));
#40423=CARTESIAN_POINT('Ctrl Pts',(1.02817560875013,0.627580438894908,56.2916035312058));
#40424=CARTESIAN_POINT('Ctrl Pts',(0.89928600670914,0.776794433451253,56.2995286529715));
#40425=CARTESIAN_POINT('Ctrl Pts',(0.77039640466815,0.926008428007598,56.3074537747372));
#40426=CARTESIAN_POINT('Ctrl Pts',(0.603569097722146,1.04245221774004,56.315378896503));
#40427=CARTESIAN_POINT('Ctrl Pts',(0.41906298399761,1.1119852356127,56.3233040182687));
#40428=CARTESIAN_POINT('Ctrl Pts',(0.234556870273075,1.18151825348535,56.3312291400344));
#40429=CARTESIAN_POINT('Ctrl Pts',(0.0323719497700094,1.20414049949823,
56.3391542618001));
#40430=CARTESIAN_POINT('Ctrl Pts',(-0.162939135811373,1.17710482606222,
56.3470793835658));
#40431=CARTESIAN_POINT('Ctrl Pts',(-0.358250221392757,1.15006915262621,
56.3550045053316));
#40432=CARTESIAN_POINT('Ctrl Pts',(-0.546687472052457,1.0733755597413,56.3629296270973));
#40433=CARTESIAN_POINT('Ctrl Pts',(-0.705367732965258,0.956337440296682,
56.370854748863));
#40434=CARTESIAN_POINT('Ctrl Pts',(-0.864047993878058,0.839299320852068,
56.3787798706287));
#40435=CARTESIAN_POINT('Ctrl Pts',(-0.992971265043959,0.681916674847751,
56.3867049923944));
#40436=CARTESIAN_POINT('Ctrl Pts',(-1.07648155278485,0.503301504297487,
56.3946301141602));
#40437=CARTESIAN_POINT('Ctrl Pts',(-1.14982814256138,0.346424860753121,
56.4015907015417));
#40438=CARTESIAN_POINT('Ctrl Pts',(-1.18814313612308,0.173169438048752,
56.4085512889233));
#40439=CARTESIAN_POINT('Ctrl Pts',(-1.18829206995915,-2.22507172762053E-5,
56.4155118763048));
#40440=CARTESIAN_POINT('Origin',(0.,0.,57.95));
#40441=CARTESIAN_POINT('',(-1.1881295160484,7.99197013834352E-6,56.7580381236952));
#40442=CARTESIAN_POINT('',(-1.18812635417301,6.58327025343463E-7,56.7155118763048));
#40443=CARTESIAN_POINT('',(-1.188225,-1.45515594291686E-16,57.95));
#40444=CARTESIAN_POINT('Ctrl Pts',(-1.1881295160484,7.99197013834352E-6,
56.7580381236952));
#40445=CARTESIAN_POINT('Ctrl Pts',(-1.18815070391462,0.0899160987151799,
56.7544261311544));
#40446=CARTESIAN_POINT('Ctrl Pts',(-1.17807704964198,0.179819532343893,
56.7508141386136));
#40447=CARTESIAN_POINT('Ctrl Pts',(-1.15785703751179,0.267379902805148,
56.7472021460728));
#40448=CARTESIAN_POINT('Ctrl Pts',(-1.11349203497487,0.459497297821303,
56.739277024307));
#40449=CARTESIAN_POINT('Ctrl Pts',(-1.02028110348739,0.640334872175578,
56.7313519025413));
#40450=CARTESIAN_POINT('Ctrl Pts',(-0.889543452490429,0.787932343460453,
56.7234267807756));
#40451=CARTESIAN_POINT('Ctrl Pts',(-0.758805801493465,0.935529814745327,
56.7155016590099));
#40452=CARTESIAN_POINT('Ctrl Pts',(-0.590541430987019,1.0498871829608,56.7075765372442));
#40453=CARTESIAN_POINT('Ctrl Pts',(-0.405183777488024,1.1171172893659,56.6996514154785));
#40454=CARTESIAN_POINT('Ctrl Pts',(-0.21982612398903,1.18434739577099,56.6917262937127));
#40455=CARTESIAN_POINT('Ctrl Pts',(-0.0173751874974873,1.2044502403657,
56.683801171947));
#40456=CARTESIAN_POINT('Ctrl Pts',(0.177584098490914,1.174984604028,56.6758760501813));
#40457=CARTESIAN_POINT('Ctrl Pts',(0.372543384479318,1.1455189676903,56.6679509284156));
#40458=CARTESIAN_POINT('Ctrl Pts',(0.56001101996458,1.06648485042019,56.6600258066499));
#40459=CARTESIAN_POINT('Ctrl Pts',(0.717221591109313,0.947479878934791,
56.6521006848842));
#40460=CARTESIAN_POINT('Ctrl Pts',(0.874432162254045,0.828474907449395,
56.6441755631184));
#40461=CARTESIAN_POINT('Ctrl Pts',(1.00138566905825,0.669499081748719,56.6362504413527));
#40462=CARTESIAN_POINT('Ctrl Pts',(1.08266532177563,0.489857869962454,56.628325319587));
#40463=CARTESIAN_POINT('Ctrl Pts',(1.16394497449302,0.310216658176189,56.6204001978213));
#40464=CARTESIAN_POINT('Ctrl Pts',(1.19955077312359,0.109910060304336,56.6124750760556));
#40465=CARTESIAN_POINT('Ctrl Pts',(1.18515887404106,-0.0867373911377846,
56.6045499542899));
#40466=CARTESIAN_POINT('Ctrl Pts',(1.17076697495852,-0.283384842579906,
56.5966248325241));
#40467=CARTESIAN_POINT('Ctrl Pts',(1.10637737816288,-0.476373147592297,
56.5886997107584));
#40468=CARTESIAN_POINT('Ctrl Pts',(0.999809331035505,-0.642266481543283,
56.5807745889927));
#40469=CARTESIAN_POINT('Ctrl Pts',(0.893241283908128,-0.808159815494271,
56.572849467227));
#40470=CARTESIAN_POINT('Ctrl Pts',(0.744494786449013,-0.946958178383857,
56.5649243454613));
#40471=CARTESIAN_POINT('Ctrl Pts',(0.571633092951576,-1.04180638257905,
56.5569992236955));
#40472=CARTESIAN_POINT('Ctrl Pts',(0.39877139945414,-1.13665458677424,56.5490741019298));
#40473=CARTESIAN_POINT('Ctrl Pts',(0.201794509918382,-1.18755263227503,
56.5411489801641));
#40474=CARTESIAN_POINT('Ctrl Pts',(0.00462260872706689,-1.18831963849283,
56.5332238583984));
#40475=CARTESIAN_POINT('Ctrl Pts',(-0.192549292464249,-1.18908664471064,
56.5252987366327));
#40476=CARTESIAN_POINT('Ctrl Pts',(-0.389916205311122,-1.13972261164545,
56.5173736148669));
#40477=CARTESIAN_POINT('Ctrl Pts',(-0.563510582363015,-1.046222134781,56.5094484931012));
#40478=CARTESIAN_POINT('Ctrl Pts',(-0.737104959414911,-0.952721657916548,
56.5015233713355));
#40479=CARTESIAN_POINT('Ctrl Pts',(-0.886926800671826,-0.815084737252838,
56.4935982495698));
#40480=CARTESIAN_POINT('Ctrl Pts',(-0.994782265853485,-0.650025518946005,
56.4856731278041));
#40481=CARTESIAN_POINT('Ctrl Pts',(-1.10263773103514,-0.484966300639175,
56.4777480060383));
#40482=CARTESIAN_POINT('Ctrl Pts',(-1.16852682014155,-0.292484784689223,
56.4698228842726));
#40483=CARTESIAN_POINT('Ctrl Pts',(-1.1844481926866,-0.0959552530276115,
56.4618977625069));
#40484=CARTESIAN_POINT('Ctrl Pts',(-1.18703283215031,-0.0640510951492984,
56.4606112162363));
#40485=CARTESIAN_POINT('Ctrl Pts',(-1.18830064548179,-0.0320402577338833,
56.4593246699657));
#40486=CARTESIAN_POINT('Ctrl Pts',(-1.18826932065667,-2.69461188108222E-5,
56.4580381236952));
#40487=CARTESIAN_POINT('Ctrl Pts',(-1.18829206995915,-2.22507172762053E-5,
56.4155118763048));
#40488=CARTESIAN_POINT('Ctrl Pts',(-1.18831270784472,-0.0240215671124719,
56.416476410689));
#40489=CARTESIAN_POINT('Ctrl Pts',(-1.1876004858046,-0.0480196596965209,
56.4174409450732));
#40490=CARTESIAN_POINT('Ctrl Pts',(-1.18614706359603,-0.0719727779040691,
56.4184054794573));
#40491=CARTESIAN_POINT('Ctrl Pts',(-1.17420498235045,-0.268784194459149,
56.426330601223));
#40492=CARTESIAN_POINT('Ctrl Pts',(-1.11222351554338,-0.462559332473099,
56.4342557229888));
#40493=CARTESIAN_POINT('Ctrl Pts',(-1.00772947510678,-0.629766816194386,
56.4421808447545));
#40494=CARTESIAN_POINT('Ctrl Pts',(-0.903235434670179,-0.796974299915674,
56.4501059665202));
#40495=CARTESIAN_POINT('Ctrl Pts',(-0.756228820604034,-0.937614129344298,
56.4580310882859));
#40496=CARTESIAN_POINT('Ctrl Pts',(-0.584561602112513,-1.03460749599802,
56.4659562100516));
#40497=CARTESIAN_POINT('Ctrl Pts',(-0.412894383620994,-1.13160086265175,
56.4738813318173));
#40498=CARTESIAN_POINT('Ctrl Pts',(-0.216566560704099,-1.18494776653058,
56.4818064535831));
#40499=CARTESIAN_POINT('Ctrl Pts',(-0.0194194972431365,-1.1881699460625,
56.4897315753488));
#40500=CARTESIAN_POINT('Ctrl Pts',(0.177727566217826,-1.19139212559442,
56.4976566971145));
#40501=CARTESIAN_POINT('Ctrl Pts',(0.375693870222856,-1.14448958077944,
56.5055818188802));
#40502=CARTESIAN_POINT('Ctrl Pts',(0.55043907930015,-1.05315799266839,56.5135069406459));
#40503=CARTESIAN_POINT('Ctrl Pts',(0.725184288377445,-0.961826404557346,
56.5214320624117));
#40504=CARTESIAN_POINT('Ctrl Pts',(0.876708402527002,-0.826065773150231,
56.5293571841774));
#40505=CARTESIAN_POINT('Ctrl Pts',(0.986610863427943,-0.662362394554791,
56.5372823059431));
#40506=CARTESIAN_POINT('Ctrl Pts',(1.09651332432888,-0.498659015959353,
56.5452074277088));
#40507=CARTESIAN_POINT('Ctrl Pts',(1.16479413198121,-0.30701289017559,56.5531325494745));
#40508=CARTESIAN_POINT('Ctrl Pts',(1.18316150395738,-0.110696852303948,
56.5610576712402));
#40509=CARTESIAN_POINT('Ctrl Pts',(1.20152887593356,0.0856191855676947,
56.568982793006));
#40510=CARTESIAN_POINT('Ctrl Pts',(1.1699828122336,0.286605135527218,56.5769079147717));
#40511=CARTESIAN_POINT('Ctrl Pts',(1.09235415648164,0.467853966927145,56.5848330365374));
#40512=CARTESIAN_POINT('Ctrl Pts',(1.01472550072968,0.649102798327074,56.5927581583031));
#40513=CARTESIAN_POINT('Ctrl Pts',(0.891014252925719,0.810614511167405,
56.6006832800688));
#40514=CARTESIAN_POINT('Ctrl Pts',(0.736243474222775,0.932775688051391,
56.6086084018345));
#40515=CARTESIAN_POINT('Ctrl Pts',(0.581472695519832,1.05493686493538,56.6165335236003));
#40516=CARTESIAN_POINT('Ctrl Pts',(0.395642385917902,1.13774750586301,56.624458645366));
#40517=CARTESIAN_POINT('Ctrl Pts',(0.201319128128168,1.17115137629747,56.6323837671317));
#40518=CARTESIAN_POINT('Ctrl Pts',(0.00699587033843588,1.20455524673192,
56.6403088888974));
#40519=CARTESIAN_POINT('Ctrl Pts',(-0.1958203356391,1.18855234667319,56.6482340106631));
#40520=CARTESIAN_POINT('Ctrl Pts',(-0.382500199260759,1.12508601232077,
56.6561591324289));
#40521=CARTESIAN_POINT('Ctrl Pts',(-0.569180062882424,1.06161967796835,
56.6640842541946));
#40522=CARTESIAN_POINT('Ctrl Pts',(-0.739723584148212,0.950689909322242,
56.6720093759603));
#40523=CARTESIAN_POINT('Ctrl Pts',(-0.873420554445836,0.80576762942286,
56.679934497726));
#40524=CARTESIAN_POINT('Ctrl Pts',(-1.00711752474346,0.660845349523481,
56.6878596194917));
#40525=CARTESIAN_POINT('Ctrl Pts',(-1.10396794407292,0.481930558370832,
56.6957847412574));
#40526=CARTESIAN_POINT('Ctrl Pts',(-1.15221063632171,0.290750042306688,
56.7037098630232));
#40527=CARTESIAN_POINT('Ctrl Pts',(-1.17615815037868,0.195848661756558,
56.7076438674504));
#40528=CARTESIAN_POINT('Ctrl Pts',(-1.18812824895107,0.0979248876013811,
56.7115778718776));
#40529=CARTESIAN_POINT('Ctrl Pts',(-1.18812635417301,6.58327025343463E-7,
56.7155118763048));
#40530=CARTESIAN_POINT('Origin',(0.,0.,57.95));
#40531=CARTESIAN_POINT('',(-1.18831370045495,1.46328030788886E-5,57.0580381236952));
#40532=CARTESIAN_POINT('',(-1.18829575305801,2.12367321252666E-5,57.0155118763048));
#40533=CARTESIAN_POINT('',(-1.188225,-1.45515594291686E-16,57.95));
#40534=CARTESIAN_POINT('Ctrl Pts',(-1.18831370045495,1.46328030788886E-5,
57.0580381236952));
#40535=CARTESIAN_POINT('Ctrl Pts',(-1.18832270521549,0.0145798869936275,
57.0574527141087));
#40536=CARTESIAN_POINT('Ctrl Pts',(-1.18806045407433,0.0291448164884335,
57.0568673045222));
#40537=CARTESIAN_POINT('Ctrl Pts',(-1.18752484989022,0.0436996868738372,
57.0562818949358));
#40538=CARTESIAN_POINT('Ctrl Pts',(-1.18027398062638,0.240739712789417,
57.0483567731701));
#40539=CARTESIAN_POINT('Ctrl Pts',(-1.12292560142346,0.435936202127469,
57.0404316514043));
#40540=CARTESIAN_POINT('Ctrl Pts',(-1.02244389883069,0.605585176076476,
57.0325065296386));
#40541=CARTESIAN_POINT('Ctrl Pts',(-0.921962196237911,0.775234150025483,
57.0245814078729));
#40542=CARTESIAN_POINT('Ctrl Pts',(-0.778347170255276,0.919335608585445,
57.0166562861072));
#40543=CARTESIAN_POINT('Ctrl Pts',(-0.609038927231272,1.02039037473736,
57.0087311643415));
#40544=CARTESIAN_POINT('Ctrl Pts',(-0.439730684207273,1.12144514088928,
57.0008060425757));
#40545=CARTESIAN_POINT('Ctrl Pts',(-0.244729224141906,1.17945321463315,
56.99288092081));
#40546=CARTESIAN_POINT('Ctrl Pts',(-0.0477148421740822,1.18737029842252,
56.9849557990443));
#40547=CARTESIAN_POINT('Ctrl Pts',(0.149299539793748,1.19528738221189,56.9770306772786));
#40548=CARTESIAN_POINT('Ctrl Pts',(0.348326843664036,1.15311347604675,56.9691055555129));
#40549=CARTESIAN_POINT('Ctrl Pts',(0.525197889909765,1.0659700315553,56.9611804337472));
#40550=CARTESIAN_POINT('Ctrl Pts',(0.702068936155495,0.978826587063846,
56.9532553119814));
#40551=CARTESIAN_POINT('Ctrl Pts',(0.856783724776667,0.846713604246079,
56.9453301902157));
#40552=CARTESIAN_POINT('Ctrl Pts',(0.970554233080142,0.685674421566015,
56.93740506845));
#40553=CARTESIAN_POINT('Ctrl Pts',(1.08432474138362,0.524635238885952,56.9294799466843));
#40554=CARTESIAN_POINT('Ctrl Pts',(1.15715096936939,0.334669856343592,56.9215548249186));
#40555=CARTESIAN_POINT('Ctrl Pts',(1.18018915467806,0.138847005441106,56.9136297031528));
#40556=CARTESIAN_POINT('Ctrl Pts',(1.20322733998672,-0.0569758454613808,
56.9057045813871));
#40557=CARTESIAN_POINT('Ctrl Pts',(1.17647748261828,-0.25865616472399,56.8977794596214));
#40558=CARTESIAN_POINT('Ctrl Pts',(1.10318799167282,-0.441702599911483,
56.8898543378557));
#40559=CARTESIAN_POINT('Ctrl Pts',(1.02989850072736,-0.624749035098976,
56.88192921609));
#40560=CARTESIAN_POINT('Ctrl Pts',(0.910069376204889,-0.789161586211348,
56.8740040943243));
#40561=CARTESIAN_POINT('Ctrl Pts',(0.758252247790524,-0.914974568204106,
56.8660789725585));
#40562=CARTESIAN_POINT('Ctrl Pts',(0.606435119376161,-1.04078755019686,
56.8581538507928));
#40563=CARTESIAN_POINT('Ctrl Pts',(0.422629987069901,-1.12800096307001,
56.8502287290271));
#40564=CARTESIAN_POINT('Ctrl Pts',(0.229157503135587,-1.16602391506192,
56.8423036072614));
#40565=CARTESIAN_POINT('Ctrl Pts',(0.0356850192012729,-1.20404686705384,
56.8343784854957));
#40566=CARTESIAN_POINT('Ctrl Pts',(-0.167454816361101,-1.19287935816454,
56.8264533637299));
#40567=CARTESIAN_POINT('Ctrl Pts',(-0.355593412562655,-1.13387753160635,
56.8185282419642));
#40568=CARTESIAN_POINT('Ctrl Pts',(-0.543732008764212,-1.07487570504817,
56.8106031201985));
#40569=CARTESIAN_POINT('Ctrl Pts',(-0.716869365604949,-0.968039560821109,
56.8026779984328));
#40570=CARTESIAN_POINT('Ctrl Pts',(-0.853980288154606,-0.826342906536414,
56.7947528766671));
#40571=CARTESIAN_POINT('Ctrl Pts',(-0.991091210704261,-0.684646252251721,
56.7868277549014));
#40572=CARTESIAN_POINT('Ctrl Pts',(-1.09217569896284,-0.508089087909396,
56.7789026331357));
#40573=CARTESIAN_POINT('Ctrl Pts',(-1.14495840629895,-0.318111897899217,
56.7709775113699));
#40574=CARTESIAN_POINT('Ctrl Pts',(-1.17368460689391,-0.214719647972578,
56.766664382145));
#40575=CARTESIAN_POINT('Ctrl Pts',(-1.18810421533032,-0.107352496286196,
56.7623512529201));
#40576=CARTESIAN_POINT('Ctrl Pts',(-1.1881295160484,7.99197013834352E-6,
56.7580381236952));
#40577=CARTESIAN_POINT('Ctrl Pts',(-1.18812635417301,6.58327025343463E-7,
56.7155118763048));
#40578=CARTESIAN_POINT('Ctrl Pts',(-1.18812443188702,-0.0993452108875006,
56.7195029936433));
#40579=CARTESIAN_POINT('Ctrl Pts',(-1.17580038004544,-0.198691548531745,
56.7234941109818));
#40580=CARTESIAN_POINT('Ctrl Pts',(-1.15115986037899,-0.294882880829771,
56.7274852283203));
#40581=CARTESIAN_POINT('Ctrl Pts',(-1.10223142701937,-0.485889046926449,
56.735410350086));
#40582=CARTESIAN_POINT('Ctrl Pts',(-1.00473959513201,-0.664455138144163,
56.7433354718517));
#40583=CARTESIAN_POINT('Ctrl Pts',(-0.870523431726741,-0.808896713041235,
56.7512605936175));
#40584=CARTESIAN_POINT('Ctrl Pts',(-0.73630726832148,-0.953338287938303,
56.7591857153832));
#40585=CARTESIAN_POINT('Ctrl Pts',(-0.565366773398321,-1.06365534651473,
56.7671108371489));
#40586=CARTESIAN_POINT('Ctrl Pts',(-0.378460362661497,-1.12645137109791,
56.7750359589146));
#40587=CARTESIAN_POINT('Ctrl Pts',(-0.191553951924672,-1.18924739568109,
56.7829610806803));
#40588=CARTESIAN_POINT('Ctrl Pts',(0.0113183746258182,-1.20452238627102,
56.7908862024461));
#40589=CARTESIAN_POINT('Ctrl Pts',(0.205520511359668,-1.1704214014468,56.7988113242118));
#40590=CARTESIAN_POINT('Ctrl Pts',(0.399722648093518,-1.13632041662258,
56.8067364459775));
#40591=CARTESIAN_POINT('Ctrl Pts',(0.58525459501073,-1.0528434563842,56.8146615677432));
#40592=CARTESIAN_POINT('Ctrl Pts',(0.739586001522012,-0.930127670756498,
56.8225866895089));
#40593=CARTESIAN_POINT('Ctrl Pts',(0.893917408033295,-0.807411885128797,
56.8305118112747));
#40594=CARTESIAN_POINT('Ctrl Pts',(1.01704827413865,-0.64545727411177,56.8384369330404));
#40595=CARTESIAN_POINT('Ctrl Pts',(1.09402601820557,-0.463931039103322,
56.8463620548061));
#40596=CARTESIAN_POINT('Ctrl Pts',(1.17100376227249,-0.282404804094877,
56.8542871765718));
#40597=CARTESIAN_POINT('Ctrl Pts',(1.20182838430099,-0.081306945095011,
56.8622122983375));
#40598=CARTESIAN_POINT('Ctrl Pts',(1.18275665002534,0.114941917397725,56.8701374201032));
#40599=CARTESIAN_POINT('Ctrl Pts',(1.16368491574969,0.311190779890463,56.878062541869));
#40600=CARTESIAN_POINT('Ctrl Pts',(1.09471682516991,0.50259064587607,56.8859876636347));
#40601=CARTESIAN_POINT('Ctrl Pts',(0.984227621935687,0.665898585201267,
56.8939127854004));
#40602=CARTESIAN_POINT('Ctrl Pts',(0.87373841870147,0.829206524526464,56.9018379071661));
#40603=CARTESIAN_POINT('Ctrl Pts',(0.721728102812821,0.964422537191249,
56.9097630289318));
#40604=CARTESIAN_POINT('Ctrl Pts',(0.546656275255271,1.05512646364228,56.9176881506976));
#40605=CARTESIAN_POINT('Ctrl Pts',(0.371584447697719,1.14583039009331,56.9256132724633));
#40606=CARTESIAN_POINT('Ctrl Pts',(0.173451108471265,1.19202223033058,56.933538394229));
#40607=CARTESIAN_POINT('Ctrl Pts',(-0.0236831228360759,1.18809260886808,
56.9414635159947));
#40608=CARTESIAN_POINT('Ctrl Pts',(-0.220817354143417,1.18416298740558,
56.9493886377604));
#40609=CARTESIAN_POINT('Ctrl Pts',(-0.416952477531646,1.1301119042433,56.9573137595261));
#40610=CARTESIAN_POINT('Ctrl Pts',(-0.588270529753804,1.03250313383418,
56.9652388812919));
#40611=CARTESIAN_POINT('Ctrl Pts',(-0.759588581975962,0.93489436342506,
56.9731640030576));
#40612=CARTESIAN_POINT('Ctrl Pts',(-0.90608956303205,0.793727905769093,
56.9810891248233));
#40613=CARTESIAN_POINT('Ctrl Pts',(-1.00998290628536,0.62614652164298,56.989014246589));
#40614=CARTESIAN_POINT('Ctrl Pts',(-1.11387624953867,0.458565137516867,
56.9969393683547));
#40615=CARTESIAN_POINT('Ctrl Pts',(-1.17516195498921,0.264568826920607,
57.0048644901205));
#40616=CARTESIAN_POINT('Ctrl Pts',(-1.18639770096215,0.0677158231578859,
57.0127896118862));
#40617=CARTESIAN_POINT('Ctrl Pts',(-1.1876841868309,0.0451762776598449,
57.0136970333591));
#40618=CARTESIAN_POINT('Ctrl Pts',(-1.18831451240506,0.0225992806104096,
57.014604454832));
#40619=CARTESIAN_POINT('Ctrl Pts',(-1.18829575305801,2.12367321252666E-5,
57.0155118763048));
#40620=CARTESIAN_POINT('Origin',(0.,0.,57.95));
#40621=CARTESIAN_POINT('',(-1.1881820096365,-2.79964409908851E-5,57.3580381236952));
#40622=CARTESIAN_POINT('',(-1.18820495619059,-3.01830341203513E-5,57.3155118763048));
#40623=CARTESIAN_POINT('',(-1.188225,-1.45515594291686E-16,57.95));
#40624=CARTESIAN_POINT('Ctrl Pts',(-1.1881820096365,-2.79964409908851E-5,
57.3580381236952));
#40625=CARTESIAN_POINT('Ctrl Pts',(-1.18806234971613,0.136458721817245,
57.3525541752973));
#40626=CARTESIAN_POINT('Ctrl Pts',(-1.1645682320165,0.272985576997064,57.3470702268995));
#40627=CARTESIAN_POINT('Ctrl Pts',(-1.11848096038993,0.401404126766149,
57.3415862785016));
#40628=CARTESIAN_POINT('Ctrl Pts',(-1.05187799242009,0.58698804733984,57.3336611567359));
#40629=CARTESIAN_POINT('Ctrl Pts',(-0.938090234140422,0.755638135133434,
57.3257360349702));
#40630=CARTESIAN_POINT('Ctrl Pts',(-0.790935672853952,0.886874113471996,
57.3178109132045));
#40631=CARTESIAN_POINT('Ctrl Pts',(-0.643781111567482,1.01811009181056,
57.3098857914388));
#40632=CARTESIAN_POINT('Ctrl Pts',(-0.463259747274216,1.11193196069409,
57.3019606696731));
#40633=CARTESIAN_POINT('Ctrl Pts',(-0.271293462938056,1.15694632058136,
57.2940355479073));
#40634=CARTESIAN_POINT('Ctrl Pts',(-0.0793271786018923,1.20196068046864,
57.2861104261416));
#40635=CARTESIAN_POINT('Ctrl Pts',(0.124084025777165,1.19816753135966,57.2781853043759));
#40636=CARTESIAN_POINT('Ctrl Pts',(0.314238605130466,1.14602750001269,57.2702601826102));
#40637=CARTESIAN_POINT('Ctrl Pts',(0.504393184483765,1.09388746866572,57.2623350608444));
#40638=CARTESIAN_POINT('Ctrl Pts',(0.681291138811312,0.993400555080754,
57.2544099390787));
#40639=CARTESIAN_POINT('Ctrl Pts',(0.823450599379697,0.856769538511313,
57.246484817313));
#40640=CARTESIAN_POINT('Ctrl Pts',(0.965610059948084,0.720138521941871,
57.2385596955473));
#40641=CARTESIAN_POINT('Ctrl Pts',(1.07303102675731,0.547363402387949,57.2306345737816));
#40642=CARTESIAN_POINT('Ctrl Pts',(1.13266867338764,0.359425385950907,57.2227094520159));
#40643=CARTESIAN_POINT('Ctrl Pts',(1.19230632001797,0.171487369513864,57.2147843302501));
#40644=CARTESIAN_POINT('Ctrl Pts',(1.20416064646939,-0.0316135438062997,
57.2068592084844));
#40645=CARTESIAN_POINT('Ctrl Pts',(1.1667921048075,-0.225213489601638,57.1989340867187));
#40646=CARTESIAN_POINT('Ctrl Pts',(1.12942356314562,-0.418813435396977,
57.191008964953));
#40647=CARTESIAN_POINT('Ctrl Pts',(1.04283215337043,-0.602912413667489,
57.1830838431873));
#40648=CARTESIAN_POINT('Ctrl Pts',(0.917533233363273,-0.755154088523403,
57.1751587214215));
#40649=CARTESIAN_POINT('Ctrl Pts',(0.792234313356116,-0.907395763379314,
57.1672335996558));
#40650=CARTESIAN_POINT('Ctrl Pts',(0.628227883116994,-1.02778013482063,
57.1593084778901));
#40651=CARTESIAN_POINT('Ctrl Pts',(0.445430309792281,-1.10168814591881,
57.1513833561244));
#40652=CARTESIAN_POINT('Ctrl Pts',(0.262632736467569,-1.17559615701699,
57.1434582343587));
#40653=CARTESIAN_POINT('Ctrl Pts',(0.0610440200572671,-1.20302780777205,
57.135533112593));
#40654=CARTESIAN_POINT('Ctrl Pts',(-0.134855610933311,-1.18065189448011,
57.1276079908272));
#40655=CARTESIAN_POINT('Ctrl Pts',(-0.330755241923892,-1.15827598118818,
57.1196828690615));
#40656=CARTESIAN_POINT('Ctrl Pts',(-0.520965787494748,-1.08609250384925,
57.1117577472958));
#40657=CARTESIAN_POINT('Ctrl Pts',(-0.68238874440318,-0.972867171432731,
57.1038326255301));
#40658=CARTESIAN_POINT('Ctrl Pts',(-0.843811701311613,-0.859641839016208,
57.0959075037643));
#40659=CARTESIAN_POINT('Ctrl Pts',(-0.976447069557621,-0.705374651522084,
57.0879823819986));
#40660=CARTESIAN_POINT('Ctrl Pts',(-1.06418807401824,-0.528799276528467,
57.0800572602329));
#40661=CARTESIAN_POINT('Ctrl Pts',(-1.14544786258642,-0.365267097628355,
57.0727175480537));
#40662=CARTESIAN_POINT('Ctrl Pts',(-1.18820080112409,-0.182600712158311,
57.0653778358744));
#40663=CARTESIAN_POINT('Ctrl Pts',(-1.18831370045495,1.46328030788886E-5,
57.0580381236952));
#40664=CARTESIAN_POINT('Ctrl Pts',(-1.18829575305801,2.12367321252666E-5,
57.0155118763048));
#40665=CARTESIAN_POINT('Ctrl Pts',(-1.18815067441569,-0.174589955388741,
57.0225295765977));
#40666=CARTESIAN_POINT('Ctrl Pts',(-1.14918402982291,-0.349263758015375,
57.0295472768905));
#40667=CARTESIAN_POINT('Ctrl Pts',(-1.07466852275288,-0.507161220676781,
57.0365649771833));
#40668=CARTESIAN_POINT('Ctrl Pts',(-0.990517812075319,-0.685475563819546,
57.044490098949));
#40669=CARTESIAN_POINT('Ctrl Pts',(-0.861030604224841,-0.84239455317589,
57.0524152207148));
#40670=CARTESIAN_POINT('Ctrl Pts',(-0.701931372739155,-0.958862495626329,
57.0603403424805));
#40671=CARTESIAN_POINT('Ctrl Pts',(-0.542832141253469,-1.07533043807677,
57.0682654642462));
#40672=CARTESIAN_POINT('Ctrl Pts',(-0.354120886132576,-1.1513473336213,
57.0761905860119));
#40673=CARTESIAN_POINT('Ctrl Pts',(-0.158714042031886,-1.17768195639405,
57.0841157077776));
#40674=CARTESIAN_POINT('Ctrl Pts',(0.0366928020688043,-1.20401657916681,
57.0920408295433));
#40675=CARTESIAN_POINT('Ctrl Pts',(0.238795235149295,-1.18066892916778,
57.0999659513091));
#40676=CARTESIAN_POINT('Ctrl Pts',(0.42305064474897,-1.11047426333603,57.1078910730748));
#40677=CARTESIAN_POINT('Ctrl Pts',(0.607306054348645,-1.04027959750429,
57.1158161948405));
#40678=CARTESIAN_POINT('Ctrl Pts',(0.773714440467504,-0.923237915839822,
57.1237413166062));
#40679=CARTESIAN_POINT('Ctrl Pts',(0.902067750839875,-0.773562350718361,
57.1316664383719));
#40680=CARTESIAN_POINT('Ctrl Pts',(1.03042106121224,-0.623886785596901,
57.1395915601377));
#40681=CARTESIAN_POINT('Ctrl Pts',(1.12071929583812,-0.441577337018447,
57.1475166819034));
#40682=CARTESIAN_POINT('Ctrl Pts',(1.16199695299385,-0.248773026647261,
57.1554418036691));
#40683=CARTESIAN_POINT('Ctrl Pts',(1.20327461014957,-0.0559687162760749,
57.1633669254348));
#40684=CARTESIAN_POINT('Ctrl Pts',(1.19553168983515,0.147330455887844,57.1712920472006));
#40685=CARTESIAN_POINT('Ctrl Pts',(1.13970846520658,0.33643654957613,57.1792171689663));
#40686=CARTESIAN_POINT('Ctrl Pts',(1.08388524057801,0.525542643264417,57.187142290732));
#40687=CARTESIAN_POINT('Ctrl Pts',(0.979981711635303,0.700455658477069,
57.1950674124977));
#40688=CARTESIAN_POINT('Ctrl Pts',(0.840615559448702,0.839934770542912,
57.2029925342634));
#40689=CARTESIAN_POINT('Ctrl Pts',(0.701249407262101,0.979413882608754,
57.2109176560291));
#40690=CARTESIAN_POINT('Ctrl Pts',(0.526420631831606,1.08345909152779,57.2188427777948));
#40691=CARTESIAN_POINT('Ctrl Pts',(0.33735982804395,1.13943551110907,57.2267678995606));
#40692=CARTESIAN_POINT('Ctrl Pts',(0.14829902425629,1.19541193069035,57.2346930213263));
#40693=CARTESIAN_POINT('Ctrl Pts',(-0.0549938078885346,1.20331956093389,
57.242618143092));
#40694=CARTESIAN_POINT('Ctrl Pts',(-0.247831498031896,1.16219812688607,
57.2505432648577));
#40695=CARTESIAN_POINT('Ctrl Pts',(-0.440669188175249,1.12107669283826,
57.2584683866234));
#40696=CARTESIAN_POINT('Ctrl Pts',(-0.623051736317142,1.0309261944991,57.2663935083891));
#40697=CARTESIAN_POINT('Ctrl Pts',(-0.772831243838051,0.902694193014421,
57.2743186301549));
#40698=CARTESIAN_POINT('Ctrl Pts',(-0.922610751358966,0.774462191529739,
57.2822437519206));
#40699=CARTESIAN_POINT('Ctrl Pts',(-1.03978721825889,0.608148686899538,
57.2901688736863));
#40700=CARTESIAN_POINT('Ctrl Pts',(-1.11013114431464,0.423950209313431,
57.298093995452));
#40701=CARTESIAN_POINT('Ctrl Pts',(-1.16166524725872,0.28900603092703,57.3038999557363));
#40702=CARTESIAN_POINT('Ctrl Pts',(-1.18806405705757,0.144462885027062,
57.3097059160205));
#40703=CARTESIAN_POINT('Ctrl Pts',(-1.18820495619059,-3.01830341203513E-5,
57.3155118763048));
#40704=CARTESIAN_POINT('Origin',(0.,0.,57.95));
#40705=CARTESIAN_POINT('',(-1.18818092497865,2.78399633203974E-5,57.6580381236952));
#40706=CARTESIAN_POINT('',(-1.18816109645034,2.38868568558623E-5,57.6155118763048));
#40707=CARTESIAN_POINT('',(-1.188225,-1.45515594291686E-16,57.95));
#40708=CARTESIAN_POINT('Ctrl Pts',(-1.18818092497865,2.78399633203974E-5,
57.6580381236952));
#40709=CARTESIAN_POINT('Ctrl Pts',(-1.18823417132103,0.0611879018643663,
57.6555807582517));
#40710=CARTESIAN_POINT('Ctrl Pts',(-1.18359441363642,0.122339960905958,
57.6531233928081));
#40711=CARTESIAN_POINT('Ctrl Pts',(-1.17419209887383,0.18275077751389,57.6506660273646));
#40712=CARTESIAN_POINT('Ctrl Pts',(-1.14386918147067,0.377578567107811,
57.6427409055989));
#40713=CARTESIAN_POINT('Ctrl Pts',(-1.06401121614902,0.564696742125061,
57.6348157838332));
#40714=CARTESIAN_POINT('Ctrl Pts',(-0.944315874851311,0.721382325984963,
57.6268906620675));
#40715=CARTESIAN_POINT('Ctrl Pts',(-0.824620533553604,0.878067909844868,
57.6189655403018));
#40716=CARTESIAN_POINT('Ctrl Pts',(-0.665087816279843,1.00432090254743,
57.611040418536));
#40717=CARTESIAN_POINT('Ctrl Pts',(-0.485090818124233,1.08480958232827,
57.6031152967703));
#40718=CARTESIAN_POINT('Ctrl Pts',(-0.305093819968621,1.16529826210911,
57.5951901750046));
#40719=CARTESIAN_POINT('Ctrl Pts',(-0.104632540931167,1.20002262896824,
57.5872650532389));
#40720=CARTESIAN_POINT('Ctrl Pts',(0.0919497025332866,1.18476587727015,
57.5793399314732));
#40721=CARTESIAN_POINT('Ctrl Pts',(0.288531945997738,1.16950912557206,57.5714148097074));
#40722=CARTESIAN_POINT('Ctrl Pts',(0.481235153889179,1.10427125531675,57.5634896879417));
#40723=CARTESIAN_POINT('Ctrl Pts',(0.646658122772754,0.996974525247105,
57.555564566176));
#40724=CARTESIAN_POINT('Ctrl Pts',(0.812081091656327,0.889677795177463,
57.5476394444103));
#40725=CARTESIAN_POINT('Ctrl Pts',(0.950223821532038,0.740322205293489,
57.5397143226446));
#40726=CARTESIAN_POINT('Ctrl Pts',(1.04431074254694,0.567044975941711,57.5317892008789));
#40727=CARTESIAN_POINT('Ctrl Pts',(1.13839766356184,0.39376774658993,57.5238640791131));
#40728=CARTESIAN_POINT('Ctrl Pts',(1.18842877571593,0.19656887777034,57.5159389573474));
#40729=CARTESIAN_POINT('Ctrl Pts',(1.18832847577251,-0.000604489746206457,
57.5080138355817));
#40730=CARTESIAN_POINT('Ctrl Pts',(1.18822817582909,-0.197777857262752,
57.500088713816));
#40731=CARTESIAN_POINT('Ctrl Pts',(1.13799646378815,-0.394925723476249,
57.4921635920503));
#40732=CARTESIAN_POINT('Ctrl Pts',(1.0437333030349,-0.568107141193917,57.4842384702846));
#40733=CARTESIAN_POINT('Ctrl Pts',(0.949470142281659,-0.741288558911583,
57.4763133485188));
#40734=CARTESIAN_POINT('Ctrl Pts',(0.811175532816112,-0.890503528133416,
57.4683882267531));
#40735=CARTESIAN_POINT('Ctrl Pts',(0.645643488217273,-0.997631904994174,
57.4604631049874));
#40736=CARTESIAN_POINT('Ctrl Pts',(0.480111443618431,-1.10476028185493,
57.4525379832217));
#40737=CARTESIAN_POINT('Ctrl Pts',(0.287341963886296,-1.16980206635462,
57.444612861456));
#40738=CARTESIAN_POINT('Ctrl Pts',(0.0907443002762212,-1.18485881171853,
57.4366877396902));
#40739=CARTESIAN_POINT('Ctrl Pts',(-0.105853363333853,-1.19991555708245,
57.4287626179245));
#40740=CARTESIAN_POINT('Ctrl Pts',(-0.306279210821867,-1.16498726331059,
57.4208374961588));
#40741=CARTESIAN_POINT('Ctrl Pts',(-0.486194228416377,-1.08431550020936,
57.4129123743931));
#40742=CARTESIAN_POINT('Ctrl Pts',(-0.666109246010887,-1.00364373710813,
57.4049872526274));
#40743=CARTESIAN_POINT('Ctrl Pts',(-0.825513433711893,-0.877228504677525,
57.3970621308616));
#40744=CARTESIAN_POINT('Ctrl Pts',(-0.945049304606873,-0.720421226506923,
57.3891370090959));
#40745=CARTESIAN_POINT('Ctrl Pts',(-1.06458517550185,-0.563613948336321,
57.3812118873302));
#40746=CARTESIAN_POINT('Ctrl Pts',(-1.14425272959081,-0.376414624425722,
57.3732867655645));
#40747=CARTESIAN_POINT('Ctrl Pts',(-1.17437741780528,-0.181556085793528,
57.3653616437988));
#40748=CARTESIAN_POINT('Ctrl Pts',(-1.18365671833321,-0.121533856599753,
57.3629204704309));
#40749=CARTESIAN_POINT('Ctrl Pts',(-1.18823527611343,-0.0607849032365112,
57.360479297063));
#40750=CARTESIAN_POINT('Ctrl Pts',(-1.1881820096365,-2.79964409908851E-5,
57.3580381236952));
#40751=CARTESIAN_POINT('Ctrl Pts',(-1.18820495619059,-3.01830341203513E-5,
57.3155118763048));
#40752=CARTESIAN_POINT('Ctrl Pts',(-1.18825638403385,-0.0527698039030566,
57.3176310377863));
#40753=CARTESIAN_POINT('Ctrl Pts',(-1.18480964802288,-0.10550275324021,
57.3197501992677));
#40754=CARTESIAN_POINT('Ctrl Pts',(-1.17781015957882,-0.157759835025051,
57.3218693607492));
#40755=CARTESIAN_POINT('Ctrl Pts',(-1.15163386357572,-0.353187951235413,
57.3297944825149));
#40756=CARTESIAN_POINT('Ctrl Pts',(-1.07576988635795,-0.541960733114136,
57.3377196042806));
#40757=CARTESIAN_POINT('Ctrl Pts',(-0.959430883924738,-0.701154274411576,
57.3456447260463));
#40758=CARTESIAN_POINT('Ctrl Pts',(-0.843091881491527,-0.860347815709018,
57.3535698478121));
#40759=CARTESIAN_POINT('Ctrl Pts',(-0.686277853842878,-0.989962116425177,
57.3614949695778));
#40760=CARTESIAN_POINT('Ctrl Pts',(-0.508031747915679,-1.07425726930934,
57.3694200913435));
#40761=CARTESIAN_POINT('Ctrl Pts',(-0.329785641988481,-1.15855242219351,
57.3773452131092));
#40762=CARTESIAN_POINT('Ctrl Pts',(-0.130107457782735,-1.19752842724568,
57.385270334875));
#40763=CARTESIAN_POINT('Ctrl Pts',(0.0667545845435723,-1.18645217476165,
57.3931954566407));
#40764=CARTESIAN_POINT('Ctrl Pts',(0.263616626869876,-1.17537592227761,
57.4011205784064));
#40765=CARTESIAN_POINT('Ctrl Pts',(0.457662527316743,-1.11424741225737,
57.4090457001721));
#40766=CARTESIAN_POINT('Ctrl Pts',(0.625328030562507,-1.0104898771126,57.4169708219378));
#40767=CARTESIAN_POINT('Ctrl Pts',(0.792993533808274,-0.90673234196783,
57.4248959437035));
#40768=CARTESIAN_POINT('Ctrl Pts',(0.934278639852939,-0.760345781698527,
57.4328210654692));
#40769=CARTESIAN_POINT('Ctrl Pts',(1.03202617967454,-0.589106868081328,
57.440746187235));
#40770=CARTESIAN_POINT('Ctrl Pts',(1.12977371949615,-0.417867954464128,
57.4486713090007));
#40771=CARTESIAN_POINT('Ctrl Pts',(1.1839836930947,-0.221776687499036,57.4565964307664));
#40772=CARTESIAN_POINT('Ctrl Pts',(1.18807303091852,-0.0246457046624006,
57.4645215525321));
#40773=CARTESIAN_POINT('Ctrl Pts',(1.19216236874234,0.172485278174231,57.4724466742978));
#40774=CARTESIAN_POINT('Ctrl Pts',(1.14613107079145,0.370655976882405,57.4803717960636));
#40775=CARTESIAN_POINT('Ctrl Pts',(1.05556901685821,0.545801235069337,57.4882969178293));
#40776=CARTESIAN_POINT('Ctrl Pts',(0.965006962924976,0.720946493256271,
57.496222039595));
#40777=CARTESIAN_POINT('Ctrl Pts',(0.829914153009402,0.873066310921964,
57.5041471613607));
#40778=CARTESIAN_POINT('Ctrl Pts',(0.666695785353968,0.983687789568155,
57.5120722831264));
#40779=CARTESIAN_POINT('Ctrl Pts',(0.503477417698534,1.09430926821435,57.5199974048921));
#40780=CARTESIAN_POINT('Ctrl Pts',(0.312133492303237,1.16343240784103,57.5279225266578));
#40781=CARTESIAN_POINT('Ctrl Pts',(0.115900146091773,1.18266313618466,57.5358476484236));
#40782=CARTESIAN_POINT('Ctrl Pts',(-0.0803332001196921,1.20189386452828,
57.5437727701893));
#40783=CARTESIAN_POINT('Ctrl Pts',(-0.281455967147326,1.17123218158885,
57.551697891955));
#40784=CARTESIAN_POINT('Ctrl Pts',(-0.463044509748822,1.09440153487909,
57.5596230137207));
#40785=CARTESIAN_POINT('Ctrl Pts',(-0.644633052350318,1.01757088816933,
57.5675481354864));
#40786=CARTESIAN_POINT('Ctrl Pts',(-0.806687370525673,0.89457127768925,
57.5754732572522));
#40787=CARTESIAN_POINT('Ctrl Pts',(-0.929528154788486,0.740339345847389,
57.5833983790179));
#40788=CARTESIAN_POINT('Ctrl Pts',(-1.0523689390513,0.58610741400553,57.5913235007836));
#40789=CARTESIAN_POINT('Ctrl Pts',(-1.13599618940157,0.400643160801886,
57.5992486225493));
#40790=CARTESIAN_POINT('Ctrl Pts',(-1.17025450510903,0.206468716337991,
57.607173744315));
#40791=CARTESIAN_POINT('Ctrl Pts',(-1.18226905691703,0.13837082901852,57.609953121645));
#40792=CARTESIAN_POINT('Ctrl Pts',(-1.18821153704315,0.0692016423874921,
57.6127324989749));
#40793=CARTESIAN_POINT('Ctrl Pts',(-1.18816109645034,2.38868568558623E-5,
57.6155118763048));
#40794=CARTESIAN_POINT('Origin',(0.,0.,57.95));
#40795=CARTESIAN_POINT('',(-1.18831445454319,-1.42653502743784E-5,57.9580381236952));
#40796=CARTESIAN_POINT('',(-1.18832572782012,-6.43342140850944E-6,57.9155118763048));
#40797=CARTESIAN_POINT('',(-1.188225,-1.45515594291686E-16,57.95));
#40798=CARTESIAN_POINT('Ctrl Pts',(-1.18831445454319,-1.42653502743784E-5,
57.9580381236952));
#40799=CARTESIAN_POINT('Ctrl Pts',(-1.18820367858962,0.183003608488043,
57.9506822194403));
#40800=CARTESIAN_POINT('Ctrl Pts',(-1.14525528855688,0.366071677622651,
57.9433263151854));
#40801=CARTESIAN_POINT('Ctrl Pts',(-1.06364953455008,0.529881684332512,
57.9359704109305));
#40802=CARTESIAN_POINT('Ctrl Pts',(-0.975728931606305,0.706367702180658,
57.9280452891648));
#40803=CARTESIAN_POINT('Ctrl Pts',(-0.842936683969155,0.860499869539008,
57.920120167399));
#40804=CARTESIAN_POINT('Ctrl Pts',(-0.681398617646076,0.973560915202376,
57.9121950456333));
#40805=CARTESIAN_POINT('Ctrl Pts',(-0.519860551322997,1.08662196086574,
57.9042699238676));
#40806=CARTESIAN_POINT('Ctrl Pts',(-0.329576666313986,1.15861188483414,
57.8963448021019));
#40807=CARTESIAN_POINT('Ctrl Pts',(-0.133654371946536,1.1807884825824,57.8884196803362));
#40808=CARTESIAN_POINT('Ctrl Pts',(0.0622679224209139,1.20296508033066,
57.8804945585704));
#40809=CARTESIAN_POINT('Ctrl Pts',(0.263828626146796,1.17532835185877,57.8725694368047));
#40810=CARTESIAN_POINT('Ctrl Pts',(0.446550912488195,1.10123440479111,57.864644315039));
#40811=CARTESIAN_POINT('Ctrl Pts',(0.629273198829594,1.02714045772345,57.8567191932733));
#40812=CARTESIAN_POINT('Ctrl Pts',(0.793157067786511,0.90658929206001,57.8487940715076));
#40813=CARTESIAN_POINT('Ctrl Pts',(0.918301035625923,0.754220219636168,
57.8408689497419));
#40814=CARTESIAN_POINT('Ctrl Pts',(1.04344500346533,0.601851147212326,57.8329438279761));
#40815=CARTESIAN_POINT('Ctrl Pts',(1.12984907018724,0.417664168028081,57.8250187062104));
#40816=CARTESIAN_POINT('Ctrl Pts',(1.16702062819532,0.224026304496317,57.8170935844447));
#40817=CARTESIAN_POINT('Ctrl Pts',(1.20419218620339,0.0303884409645555,
57.809168462679));
#40818=CARTESIAN_POINT('Ctrl Pts',(1.19213123549764,-0.172700306914724,
57.8012433409133));
#40819=CARTESIAN_POINT('Ctrl Pts',(1.13230241573907,-0.360577552062159,
57.7933182191476));
#40820=CARTESIAN_POINT('Ctrl Pts',(1.0724735959805,-0.548454797209594,57.7853930973818));
#40821=CARTESIAN_POINT('Ctrl Pts',(0.96487690716912,-0.721120539625185,
57.7774679756161));
#40822=CARTESIAN_POINT('Ctrl Pts',(0.822578514789886,-0.857606855584618,
57.7695428538504));
#40823=CARTESIAN_POINT('Ctrl Pts',(0.680280122410652,-0.994093171544052,
57.7616177320847));
#40824=CARTESIAN_POINT('Ctrl Pts',(0.503280026463566,-1.09440006104733,
57.753692610319));
#40825=CARTESIAN_POINT('Ctrl Pts',(0.313072499402984,-1.14634660633564,
57.7457674885532));
#40826=CARTESIAN_POINT('Ctrl Pts',(0.122864972342397,-1.19829315162395,
57.7378423667875));
#40827=CARTESIAN_POINT('Ctrl Pts',(-0.0805499858316875,-1.2018793526973,
57.7299172450218));
#40828=CARTESIAN_POINT('Ctrl Pts',(-0.27247037420288,-1.1566697138429,57.7219921232561));
#40829=CARTESIAN_POINT('Ctrl Pts',(-0.464390762574071,-1.1114600749885,
57.7140670014904));
#40830=CARTESIAN_POINT('Ctrl Pts',(-0.64481658114237,-1.01745459620635,
57.7061418797247));
#40831=CARTESIAN_POINT('Ctrl Pts',(-0.791837549682469,-0.886068973981448,
57.6982167579589));
#40832=CARTESIAN_POINT('Ctrl Pts',(-0.938858518222567,-0.754683351756544,
57.6902916361932));
#40833=CARTESIAN_POINT('Ctrl Pts',(-1.05247463673446,-0.585917586088883,
57.6823665144275));
#40834=CARTESIAN_POINT('Ctrl Pts',(-1.11888876124807,-0.400266001169753,
57.6744413926618));
#40835=CARTESIAN_POINT('Ctrl Pts',(-1.16470966595187,-0.272179940516427,
57.6689736363396));
#40836=CARTESIAN_POINT('Ctrl Pts',(-1.18806244930546,-0.136056239841935,
57.6635058800174));
#40837=CARTESIAN_POINT('Ctrl Pts',(-1.18818092497865,2.78399633203974E-5,
57.6580381236952));
#40838=CARTESIAN_POINT('Ctrl Pts',(-1.18816109645034,2.38868568558623E-5,
57.6155118763048));
#40839=CARTESIAN_POINT('Ctrl Pts',(-1.18806771064159,-0.128051940332391,
57.6206576207406));
#40840=CARTESIAN_POINT('Ctrl Pts',(-1.16743245670349,-0.256157139044143,
57.6258033651764));
#40841=CARTESIAN_POINT('Ctrl Pts',(-1.12675762900519,-0.377547590421175,
57.6309491096122));
#40842=CARTESIAN_POINT('Ctrl Pts',(-1.06411305612924,-0.56450481699229,
57.6388742313779));
#40843=CARTESIAN_POINT('Ctrl Pts',(-0.953934529312678,-0.735534634410373,
57.6467993531436));
#40844=CARTESIAN_POINT('Ctrl Pts',(-0.809601743415808,-0.869867779959869,
57.6547244749094));
#40845=CARTESIAN_POINT('Ctrl Pts',(-0.665268957518935,-1.00420092550937,
57.6626495966751));
#40846=CARTESIAN_POINT('Ctrl Pts',(-0.486781912541746,-1.10183739919028,
57.6705747184408));
#40847=CARTESIAN_POINT('Ctrl Pts',(-0.295815450827041,-1.15092056919938,
57.6784998402065));
#40848=CARTESIAN_POINT('Ctrl Pts',(-0.104848989112345,-1.20000373920847,
57.6864249619722));
#40849=CARTESIAN_POINT('Ctrl Pts',(0.0985968893398703,-1.20053360554576,
57.6943500837379));
#40850=CARTESIAN_POINT('Ctrl Pts',(0.289816428762806,-1.15244582309686,
57.7022752055036));
#40851=CARTESIAN_POINT('Ctrl Pts',(0.481035968185751,-1.10435804064796,
57.7102003272694));
#40852=CARTESIAN_POINT('Ctrl Pts',(0.660029168579411,-1.00765260941287,
57.7181254490351));
#40853=CARTESIAN_POINT('Ctrl Pts',(0.805059721857905,-0.874073098657258,
57.7260505708008));
#40854=CARTESIAN_POINT('Ctrl Pts',(0.950090275136396,-0.740493587901643,
57.7339756925665));
#40855=CARTESIAN_POINT('Ctrl Pts',(1.06115818129972,-0.5700399976255,57.7419008143322));
#40856=CARTESIAN_POINT('Ctrl Pts',(1.124775742371,-0.383411615536077,57.749825936098));
#40857=CARTESIAN_POINT('Ctrl Pts',(1.18839330344229,-0.196783233446657,
57.7577510578637));
#40858=CARTESIAN_POINT('Ctrl Pts',(1.20456051942155,0.0060199404560462,
57.7656761796294));
#40859=CARTESIAN_POINT('Ctrl Pts',(1.17131410015784,0.200370198197361,57.7736013013951));
#40860=CARTESIAN_POINT('Ctrl Pts',(1.13806768089414,0.394720455938679,57.7815264231608));
#40861=CARTESIAN_POINT('Ctrl Pts',(1.05540762638747,0.580617797518612,57.7894515449266));
#40862=CARTESIAN_POINT('Ctrl Pts',(0.93337188448839,0.735487500098281,57.7973766666923));
#40863=CARTESIAN_POINT('Ctrl Pts',(0.811336142589308,0.890357202677951,
57.805301788458));
#40864=CARTESIAN_POINT('Ctrl Pts',(0.649924713297808,1.01419926625736,57.8132269102237));
#40865=CARTESIAN_POINT('Ctrl Pts',(0.468738835923253,1.09197474387073,57.8211520319894));
#40866=CARTESIAN_POINT('Ctrl Pts',(0.287552958548701,1.1697502214841,57.8290771537551));
#40867=CARTESIAN_POINT('Ctrl Pts',(0.0865926330910932,1.20145911313143,
57.8370022755208));
#40868=CARTESIAN_POINT('Ctrl Pts',(-0.109738221543257,1.18325080193793,
57.8449273972866));
#40869=CARTESIAN_POINT('Ctrl Pts',(-0.30606907617761,1.16504249074443,57.8528525190523));
#40870=CARTESIAN_POINT('Ctrl Pts',(-0.4977704599887,1.09691697671011,57.860777640818));
#40871=CARTESIAN_POINT('Ctrl Pts',(-0.661562827553329,0.987147183936556,
57.8687027625837));
#40872=CARTESIAN_POINT('Ctrl Pts',(-0.82535519511796,0.877377391163003,
57.8766278843495));
#40873=CARTESIAN_POINT('Ctrl Pts',(-0.961238546436123,0.725963319650224,
57.8845530061152));
#40874=CARTESIAN_POINT('Ctrl Pts',(-1.05271168268295,0.551292164552578,
57.8924781278809));
#40875=CARTESIAN_POINT('Ctrl Pts',(-1.14133152854122,0.382069467313122,
57.9001560440222));
#40876=CARTESIAN_POINT('Ctrl Pts',(-1.18826849441849,0.191017958341526,
57.9078339601635));
#40877=CARTESIAN_POINT('Ctrl Pts',(-1.18832572782012,-6.43342140850944E-6,
57.9155118763048));
#40878=CARTESIAN_POINT('Origin',(0.,0.,57.95));
#40879=CARTESIAN_POINT('',(-1.18812981577958,-8.35218226485912E-6,58.2580381236952));
#40880=CARTESIAN_POINT('',(-1.18813848747178,-1.51983744768193E-5,58.2155118763048));
#40881=CARTESIAN_POINT('',(-1.188225,-1.45515594291686E-16,57.95));
#40882=CARTESIAN_POINT('Ctrl Pts',(-1.18812981577958,-8.35218226485912E-6,
58.2580381236952));
#40883=CARTESIAN_POINT('Ctrl Pts',(-1.18810326726687,0.107755104213723,
58.2537088023946));
#40884=CARTESIAN_POINT('Ctrl Pts',(-1.17357378535918,0.215525578981994,
58.2493794810941));
#40885=CARTESIAN_POINT('Ctrl Pts',(-1.14463417372155,0.319276588694579,
58.2450501597935));
#40886=CARTESIAN_POINT('Ctrl Pts',(-1.09165821509935,0.509199980423857,
58.2371250380278));
#40887=CARTESIAN_POINT('Ctrl Pts',(-0.990394153790361,0.685654212264053,
58.229199916262));
#40888=CARTESIAN_POINT('Ctrl Pts',(-0.853139143149014,0.827211299588345,
58.2212747944963));
#40889=CARTESIAN_POINT('Ctrl Pts',(-0.715884132507665,0.968768386912637,
58.2133496727306));
#40890=CARTESIAN_POINT('Ctrl Pts',(-0.542638172533966,1.07542832972103,
58.2054245509649));
#40891=CARTESIAN_POINT('Ctrl Pts',(-0.354439646542703,1.13423871768616,
58.1974994291992));
#40892=CARTESIAN_POINT('Ctrl Pts',(-0.16624112055144,1.1930491056513,58.1895743074335));
#40893=CARTESIAN_POINT('Ctrl Pts',(0.0369099714573795,1.20400993877317,
58.1816491856678));
#40894=CARTESIAN_POINT('Ctrl Pts',(0.230343671551399,1.16579017182162,58.173724063902));
#40895=CARTESIAN_POINT('Ctrl Pts',(0.423777371645419,1.12757040487008,58.1657989421363));
#40896=CARTESIAN_POINT('Ctrl Pts',(0.607493679824638,1.0401700378451,58.1578738203706));
#40897=CARTESIAN_POINT('Ctrl Pts',(0.759182730316479,0.914202665566497,
58.1499486986049));
#40898=CARTESIAN_POINT('Ctrl Pts',(0.910871780808321,0.788235293287889,
58.1420235768392));
#40899=CARTESIAN_POINT('Ctrl Pts',(1.03053357361278,0.623700915755645,58.1340984550734));
#40900=CARTESIAN_POINT('Ctrl Pts',(1.10363679922321,0.440580012188506,58.1261733333077));
#40901=CARTESIAN_POINT('Ctrl Pts',(1.17674002483363,0.257459108621373,58.118248211542));
#40902=CARTESIAN_POINT('Ctrl Pts',(1.20328468325001,0.0557516790193457,
58.1103230897763));
#40903=CARTESIAN_POINT('Ctrl Pts',(1.18004728401516,-0.140047631997551,
58.1023979680106));
#40904=CARTESIAN_POINT('Ctrl Pts',(1.1568098847803,-0.335846943014454,58.0944728462449));
#40905=CARTESIAN_POINT('Ctrl Pts',(1.0837904278942,-0.525738135446225,58.0865477244791));
#40906=CARTESIAN_POINT('Ctrl Pts',(0.969856140757953,-0.686661487178189,
58.0786226027134));
#40907=CARTESIAN_POINT('Ctrl Pts',(0.855921853621706,-0.847584838910152,
58.0706974809477));
#40908=CARTESIAN_POINT('Ctrl Pts',(0.701072736235314,-0.979540349942306,
58.062772359182));
#40909=CARTESIAN_POINT('Ctrl Pts',(0.524113123707244,-1.0665038046334,58.0548472374163));
#40910=CARTESIAN_POINT('Ctrl Pts',(0.347153511179174,-1.15346725932448,
58.0469221156505));
#40911=CARTESIAN_POINT('Ctrl Pts',(0.148083403509426,-1.19543865767451,
58.0389969938848));
#40912=CARTESIAN_POINT('Ctrl Pts',(-0.0489228218313184,-1.18732113989591,
58.0310718721191));
#40913=CARTESIAN_POINT('Ctrl Pts',(-0.245929047172062,-1.17920362211732,
58.0231467503534));
#40914=CARTESIAN_POINT('Ctrl Pts',(-0.440871390183802,-1.12099718821011,
58.0152216285877));
#40915=CARTESIAN_POINT('Ctrl Pts',(-0.610076734695811,-1.01977022388505,
58.007296506822));
#40916=CARTESIAN_POINT('Ctrl Pts',(-0.779282079207818,-0.918543259559998,
57.9993713850562));
#40917=CARTESIAN_POINT('Ctrl Pts',(-0.922750425220095,-0.774295764817101,
57.9914462632905));
#40918=CARTESIAN_POINT('Ctrl Pts',(-1.02305947868662,-0.604544650798541,
57.9835211415248));
#40919=CARTESIAN_POINT('Ctrl Pts',(-1.12336853215315,-0.434793536779981,
57.9755960197591));
#40920=CARTESIAN_POINT('Ctrl Pts',(-1.18051829307393,-0.239538803485758,
57.9676708979934));
#40921=CARTESIAN_POINT('Ctrl Pts',(-1.1875686944091,-0.0424915026696703,
57.9597457762276));
#40922=CARTESIAN_POINT('Ctrl Pts',(-1.18807508560623,-0.0283386886939873,
57.9591765587168));
#40923=CARTESIAN_POINT('Ctrl Pts',(-1.18832302665212,-0.0141766273077396,
57.958607341206));
#40924=CARTESIAN_POINT('Ctrl Pts',(-1.18831445454319,-1.42653502743784E-5,
57.9580381236952));
#40925=CARTESIAN_POINT('Ctrl Pts',(-1.18832572782012,-6.43342140850944E-6,
57.9155118763048));
#40926=CARTESIAN_POINT('Ctrl Pts',(-1.18832757056215,-0.00615683975214519,
57.9157590819292));
#40927=CARTESIAN_POINT('Ctrl Pts',(-1.18828081567409,-0.012307217971969,
57.9160062875536));
#40928=CARTESIAN_POINT('Ctrl Pts',(-1.18818528970154,-0.0184568385994857,
57.916253493178));
#40929=CARTESIAN_POINT('Ctrl Pts',(-1.18512283929783,-0.215606447971398,
57.9241786149437));
#40930=CARTESIAN_POINT('Ctrl Pts',(-1.13193501731493,-0.411977428032717,
57.9321037367095));
#40931=CARTESIAN_POINT('Ctrl Pts',(-1.03508076678807,-0.583723173927203,
57.9400288584752));
#40932=CARTESIAN_POINT('Ctrl Pts',(-0.938226516261208,-0.755468919821696,
57.9479539802409));
#40933=CARTESIAN_POINT('Ctrl Pts',(-0.797705837190388,-0.902589431549353,
57.9558791020066));
#40934=CARTESIAN_POINT('Ctrl Pts',(-0.630583069260051,-1.00721890883601,
57.9638042237723));
#40935=CARTESIAN_POINT('Ctrl Pts',(-0.463460301329717,-1.11184838612266,
57.9717293455381));
#40936=CARTESIAN_POINT('Ctrl Pts',(-0.269735444539866,-1.17398682896832,
57.9796544673038));
#40937=CARTESIAN_POINT('Ctrl Pts',(-0.0729337677935576,-1.18608836225201,
57.9875795890695));
#40938=CARTESIAN_POINT('Ctrl Pts',(0.123867908952751,-1.19818989553571,
57.9955047108352));
#40939=CARTESIAN_POINT('Ctrl Pts',(0.323746405655516,-1.16025451925745,
58.0034298326009));
#40940=CARTESIAN_POINT('Ctrl Pts',(0.502429176907867,-1.07688897280356,
58.0113549543667));
#40941=CARTESIAN_POINT('Ctrl Pts',(0.681111948160215,-0.993523426349675,
58.0192800761324));
#40942=CARTESIAN_POINT('Ctrl Pts',(0.838598993962152,-0.864727709720157,
58.0272051978981));
#40943=CARTESIAN_POINT('Ctrl Pts',(0.955765638406653,-0.706142324177889,
58.0351303196638));
#40944=CARTESIAN_POINT('Ctrl Pts',(1.07293228285115,-0.547556938635621,
58.0430554414295));
#40945=CARTESIAN_POINT('Ctrl Pts',(1.14977852593822,-0.359181884180608,
58.0509805631953));
#40946=CARTESIAN_POINT('Ctrl Pts',(1.17697242873772,-0.163892768435502,
58.058905684961));
#40947=CARTESIAN_POINT('Ctrl Pts',(1.20416633153722,0.0313963473096032,
58.0668308067267));
#40948=CARTESIAN_POINT('Ctrl Pts',(1.18170789404915,0.2335995243448,58.0747559284924));
#40949=CARTESIAN_POINT('Ctrl Pts',(1.11232439035596,0.418161916216034,58.0826810502581));
#40950=CARTESIAN_POINT('Ctrl Pts',(1.04294088666277,0.60272430808727,58.0906061720238));
#40951=CARTESIAN_POINT('Ctrl Pts',(0.926632316764456,0.769645914794549,
58.0985312937895));
#40952=CARTESIAN_POINT('Ctrl Pts',(0.777522786508502,0.898656360359332,
58.1064564155553));
#40953=CARTESIAN_POINT('Ctrl Pts',(0.628413256252548,1.02766680592411,58.114381537321));
#40954=CARTESIAN_POINT('Ctrl Pts',(0.446502765638955,1.1187660903464,58.1223066590867));
#40955=CARTESIAN_POINT('Ctrl Pts',(0.253881888272399,1.16089143521755,58.1302317808524));
#40956=CARTESIAN_POINT('Ctrl Pts',(0.0612610109058417,1.20301678008871,
58.1381569026181));
#40957=CARTESIAN_POINT('Ctrl Pts',(-0.142070253213676,1.19616818540873,
58.1460820243839));
#40958=CARTESIAN_POINT('Ctrl Pts',(-0.331420066682969,1.14117732055719,
58.1540071461496));
#40959=CARTESIAN_POINT('Ctrl Pts',(-0.520769880152256,1.08618645570565,
58.1619322679153));
#40960=CARTESIAN_POINT('Ctrl Pts',(-0.696138242971318,0.983053320682559,
58.169857389681));
#40961=CARTESIAN_POINT('Ctrl Pts',(-0.836229034648592,0.844302042615622,
58.1777825114468));
#40962=CARTESIAN_POINT('Ctrl Pts',(-0.976319826325865,0.705550764548685,
58.1857076332125));
#40963=CARTESIAN_POINT('Ctrl Pts',(-1.08113304686135,0.531181343437903,
58.1936327549782));
#40964=CARTESIAN_POINT('Ctrl Pts',(-1.13794054542014,0.342368591788372,
58.2015578767439));
#40965=CARTESIAN_POINT('Ctrl Pts',(-1.17128143419471,0.231552500397665,
58.2062092099309));
#40966=CARTESIAN_POINT('Ctrl Pts',(-1.18808611145214,0.115761211072918,
58.2108605431178));
#40967=CARTESIAN_POINT('Ctrl Pts',(-1.18813848747178,-1.51983744768193E-5,
58.2155118763048));
#40968=CARTESIAN_POINT('Origin',(0.,0.,57.95));
#40969=CARTESIAN_POINT('',(-1.18826810796675,2.71338473248756E-5,58.5580381236952));
#40970=CARTESIAN_POINT('',(-1.18824324986219,2.98497152091627E-5,58.5155118763048));
#40971=CARTESIAN_POINT('',(-1.188225,-1.45515594291686E-16,57.95));
#40972=CARTESIAN_POINT('Ctrl Pts',(-1.18826810796675,2.71338473248756E-5,
58.5580381236952));
#40973=CARTESIAN_POINT('Ctrl Pts',(-1.18829995724248,0.0324434506831562,
58.5567353853489));
#40974=CARTESIAN_POINT('Ctrl Pts',(-1.18699999162847,0.06485722040431,58.5554326470027));
#40975=CARTESIAN_POINT('Ctrl Pts',(-1.18434995694146,0.0971602348310493,
58.5541299086565));
#40976=CARTESIAN_POINT('Ctrl Pts',(-1.16822864782457,0.293673466727152,
58.5462047868908));
#40977=CARTESIAN_POINT('Ctrl Pts',(-1.1021437663709,0.486087848960798,58.538279665125));
#40978=CARTESIAN_POINT('Ctrl Pts',(-0.994120429400183,0.651037252074617,
58.5303545433593));
#40979=CARTESIAN_POINT('Ctrl Pts',(-0.886097092429467,0.815986655188435,
58.5224294215936));
#40980=CARTESIAN_POINT('Ctrl Pts',(-0.736135299941706,0.953471079182426,
58.5145042998279));
#40981=CARTESIAN_POINT('Ctrl Pts',(-0.562445887406952,1.04679489656698,
58.5065791780622));
#40982=CARTESIAN_POINT('Ctrl Pts',(-0.388756474872198,1.14011871395154,
58.4986540562965));
#40983=CARTESIAN_POINT('Ctrl Pts',(-0.191339442290451,1.18928192472666,
58.4907289345308));
#40984=CARTESIAN_POINT('Ctrl Pts',(0.00583157652335925,1.18831432056292,
58.4828038127651));
#40985=CARTESIAN_POINT('Ctrl Pts',(0.203002595337164,1.18734671639919,58.4748786909993));
#40986=CARTESIAN_POINT('Ctrl Pts',(0.399927600383042,1.1362482972966,58.4669535692336));
#40987=CARTESIAN_POINT('Ctrl Pts',(0.572692707948748,1.04122427651395,58.4590284474679));
#40988=CARTESIAN_POINT('Ctrl Pts',(0.745457815514457,0.946200255731301,
58.4511033257021));
#40989=CARTESIAN_POINT('Ctrl Pts',(0.894063025599998,0.807250633268592,
58.4431782039364));
#40990=CARTESIAN_POINT('Ctrl Pts',(1.00046224135654,0.641248965191775,58.4352530821707));
#40991=CARTESIAN_POINT('Ctrl Pts',(1.10686145711308,0.475247297114954,58.427327960405));
#40992=CARTESIAN_POINT('Ctrl Pts',(1.17105467854062,0.282193583424028,58.4194028386393));
#40993=CARTESIAN_POINT('Ctrl Pts',(1.18524650539542,0.0855315917519751,
58.4114777168736));
#40994=CARTESIAN_POINT('Ctrl Pts',(1.19943833225021,-0.111130399920075,
58.4035525951079));
#40995=CARTESIAN_POINT('Ctrl Pts',(1.16362876453227,-0.31140066957325,58.3956274733421));
#40996=CARTESIAN_POINT('Ctrl Pts',(1.08216639087305,-0.490959096264115,
58.3877023515764));
#40997=CARTESIAN_POINT('Ctrl Pts',(1.00070401721382,-0.670517522954981,
58.3797772298107));
#40998=CARTESIAN_POINT('Ctrl Pts',(0.873588837613317,-0.829364106683535,
58.371852108045));
#40999=CARTESIAN_POINT('Ctrl Pts',(0.716257274796604,-0.948209074013012,
58.3639269862793));
#41000=CARTESIAN_POINT('Ctrl Pts',(0.558925711979891,-1.06705404134249,
58.3560018645135));
#41001=CARTESIAN_POINT('Ctrl Pts',(0.371377765946969,-1.14589739227289,
58.3480767427478));
#41002=CARTESIAN_POINT('Ctrl Pts',(0.176388603167195,-1.17516466608403,
58.3401516209821));
#41003=CARTESIAN_POINT('Ctrl Pts',(-0.0186005596125763,-1.20443193989518,
58.3322264992164));
#41004=CARTESIAN_POINT('Ctrl Pts',(-0.2210309391392,-1.18412313658707,58.3243013774507));
#41005=CARTESIAN_POINT('Ctrl Pts',(-0.406320098282897,-1.11670448618739,
58.316376255685));
#41006=CARTESIAN_POINT('Ctrl Pts',(-0.591609257426595,-1.04928583578771,
58.3084511339192));
#41007=CARTESIAN_POINT('Ctrl Pts',(-0.759757196187365,-0.934757338296458,
58.3005260121535));
#41008=CARTESIAN_POINT('Ctrl Pts',(-0.890344617112157,-0.787026933795204,
58.2926008903878));
#41009=CARTESIAN_POINT('Ctrl Pts',(-1.02093203803695,-0.639296529293947,
58.2846757686221));
#41010=CARTESIAN_POINT('Ctrl Pts',(-1.11395894112576,-0.458364217782691,
58.2767506468564));
#41011=CARTESIAN_POINT('Ctrl Pts',(-1.15812846470246,-0.266201786217879,
58.2688255250906));
#41012=CARTESIAN_POINT('Ctrl Pts',(-1.17816914017951,-0.179013503030185,
58.2652297246255));
#41013=CARTESIAN_POINT('Ctrl Pts',(-1.18815186615369,-0.0895133484008016,
58.2616339241603));
#41014=CARTESIAN_POINT('Ctrl Pts',(-1.18812981577958,-8.35218226485912E-6,
58.2580381236952));
#41015=CARTESIAN_POINT('Ctrl Pts',(-1.18813848747178,-1.51983744768193E-5,
58.2155118763048));
#41016=CARTESIAN_POINT('Ctrl Pts',(-1.18817535174446,-0.0815031227393336,
58.2187856648836));
#41017=CARTESIAN_POINT('Ctrl Pts',(-1.17991331027786,-0.162983675776645,
58.2220594534623));
#41018=CARTESIAN_POINT('Ctrl Pts',(-1.16327701820942,-0.242716947204002,
58.2253332420411));
#41019=CARTESIAN_POINT('Ctrl Pts',(-1.12300421585783,-0.435733652358568,
58.2332583638068));
#41020=CARTESIAN_POINT('Ctrl Pts',(-1.03365683457257,-0.61851098047942,
58.2411834855725));
#41021=CARTESIAN_POINT('Ctrl Pts',(-0.906084907773975,-0.768853092247442,
58.2491086073382));
#41022=CARTESIAN_POINT('Ctrl Pts',(-0.778512980975379,-0.919195204015464,
58.2570337291039));
#41023=CARTESIAN_POINT('Ctrl Pts',(-0.612716508663446,-1.03710209943066,
58.2649588508696));
#41024=CARTESIAN_POINT('Ctrl Pts',(-0.428829234431794,-1.10825557758618,
58.2728839726354));
#41025=CARTESIAN_POINT('Ctrl Pts',(-0.244941960200139,-1.17940905574169,
58.2808090944011));
#41026=CARTESIAN_POINT('Ctrl Pts',(-0.0429638840487702,-1.20380911663754,
58.2887342161668));
#41027=CARTESIAN_POINT('Ctrl Pts',(0.152577483032149,-1.17849270223697,
58.2966593379325));
#41028=CARTESIAN_POINT('Ctrl Pts',(0.348118850113065,-1.15317628783641,
58.3045844596982));
#41029=CARTESIAN_POINT('Ctrl Pts',(0.537223508123526,-1.07814339813944,
58.312509581464));
#41030=CARTESIAN_POINT('Ctrl Pts',(0.69692724893745,-0.962505764784142,
58.3204347032297));
#41031=CARTESIAN_POINT('Ctrl Pts',(0.856630989751369,-0.846868131428849,
58.3283598249954));
#41032=CARTESIAN_POINT('Ctrl Pts',(0.986933813368754,-0.690625754415232,
58.3362849467611));
#41033=CARTESIAN_POINT('Ctrl Pts',(1.07201220072642,-0.512752161426865,
58.3442100685268));
#41034=CARTESIAN_POINT('Ctrl Pts',(1.15709058808409,-0.334878568438493,
58.3521351902925));
#41035=CARTESIAN_POINT('Ctrl Pts',(1.19694453918204,-0.135373759475367,
58.3600603120583));
#41036=CARTESIAN_POINT('Ctrl Pts',(1.18673432961957,0.0615350993874707,
58.367985433824));
#41037=CARTESIAN_POINT('Ctrl Pts',(1.17652412005709,0.258443958250309,58.3759105555897));
#41038=CARTESIAN_POINT('Ctrl Pts',(1.11624974983419,0.452756867012861,58.3838356773554));
#41039=CARTESIAN_POINT('Ctrl Pts',(1.01323072761359,0.620877145797678,58.3917607991211));
#41040=CARTESIAN_POINT('Ctrl Pts',(0.910211705392977,0.788997424582495,
58.3996859208868));
#41041=CARTESIAN_POINT('Ctrl Pts',(0.764448031174658,0.930925073389578,
58.4076110426526));
#41042=CARTESIAN_POINT('Ctrl Pts',(0.593640735632269,1.0294248950517,58.4155361644183));
#41043=CARTESIAN_POINT('Ctrl Pts',(0.422833440089881,1.12792471671382,58.423461286184));
#41044=CARTESIAN_POINT('Ctrl Pts',(0.226982523223422,1.18299671123099,58.4313864079497));
#41045=CARTESIAN_POINT('Ctrl Pts',(0.0298714352340844,1.18795312824677,
58.4393115297154));
#41046=CARTESIAN_POINT('Ctrl Pts',(-0.167239652755254,1.19290954526255,
58.4472366514811));
#41047=CARTESIAN_POINT('Ctrl Pts',(-0.365610911867472,1.14775038477695,
58.4551617732469));
#41048=CARTESIAN_POINT('Ctrl Pts',(-0.54115283035594,1.05795961725955,58.4630868950126));
#41049=CARTESIAN_POINT('Ctrl Pts',(-0.716694748844407,0.968168849742159,
58.4710120167783));
#41050=CARTESIAN_POINT('Ctrl Pts',(-0.869407326709119,0.833746475192972,
58.478937138544));
#41051=CARTESIAN_POINT('Ctrl Pts',(-0.9807456827269,0.671016276528948,58.4868622603097));
#41052=CARTESIAN_POINT('Ctrl Pts',(-1.09208403874468,0.508286077864927,
58.4947873820755));
#41053=CARTESIAN_POINT('Ctrl Pts',(-1.16204817291552,0.317248055086073,
58.5027125038412));
#41054=CARTESIAN_POINT('Ctrl Pts',(-1.18214188554047,0.121101197372472,
58.5106376256069));
#41055=CARTESIAN_POINT('Ctrl Pts',(-1.18626135085938,0.0808886098409063,
58.5122623758395));
#41056=CARTESIAN_POINT('Ctrl Pts',(-1.18828475300578,0.0404612970186917,
58.5138871260722));
#41057=CARTESIAN_POINT('Ctrl Pts',(-1.18824324986219,2.98497152091627E-5,
58.5155118763048));
#41058=CARTESIAN_POINT('Origin',(0.,0.,57.95));
#41059=CARTESIAN_POINT('',(-1.18823546047583,-3.02886631483035E-5,58.8580381236952));
#41060=CARTESIAN_POINT('',(-1.1882605894663,-2.81773776290431E-5,58.8155118763048));
#41061=CARTESIAN_POINT('',(-1.188225,-1.45515594291686E-16,57.95));
#41062=CARTESIAN_POINT('Ctrl Pts',(-1.18823546047583,-3.02886631483035E-5,
58.8580381236952));
#41063=CARTESIAN_POINT('Ctrl Pts',(-1.18807696349612,0.154289641889854,
58.8518368465376));
#41064=CARTESIAN_POINT('Ctrl Pts',(-1.15786515478889,0.308669815085824,
58.84563556938));
#41065=CARTESIAN_POINT('Ctrl Pts',(-1.09925951056845,0.451390584931154,
58.8394342922223));
#41066=CARTESIAN_POINT('Ctrl Pts',(-1.02436254099252,0.633785187006535,
58.8315091704566));
#41067=CARTESIAN_POINT('Ctrl Pts',(-0.90309166668407,0.797137202885021,
58.8235840486909));
#41068=CARTESIAN_POINT('Ctrl Pts',(-0.750173598378564,0.921609735210858,
58.8156589269252));
#41069=CARTESIAN_POINT('Ctrl Pts',(-0.597255530073064,1.04608226753669,
58.8077338051595));
#41070=CARTESIAN_POINT('Ctrl Pts',(-0.412690267770512,1.13167531630988,
58.7998086833938));
#41071=CARTESIAN_POINT('Ctrl Pts',(-0.218890771262336,1.16799476111661,
58.791883561628));
#41072=CARTESIAN_POINT('Ctrl Pts',(-0.0250912747541551,1.20431420592335,
58.7839584398623));
#41073=CARTESIAN_POINT('Ctrl Pts',(0.17794245595965,1.19136004676362,58.7760333180966));
#41074=CARTESIAN_POINT('Ctrl Pts',(0.365554714891826,1.1307053914084,58.7681081963309));
#41075=CARTESIAN_POINT('Ctrl Pts',(0.553166973824001,1.07005073605319,58.7601830745652));
#41076=CARTESIAN_POINT('Ctrl Pts',(0.725357760974547,0.961695584502476,
58.7522579527995));
#41077=CARTESIAN_POINT('Ctrl Pts',(0.861216829525005,0.818798207302978,
58.7443328310337));
#41078=CARTESIAN_POINT('Ctrl Pts',(0.997075898075464,0.67590083010348,58.736407709268));
#41079=CARTESIAN_POINT('Ctrl Pts',(1.09660324802584,0.498461227255193,58.7284825875023));
#41080=CARTESIAN_POINT('Ctrl Pts',(1.14771262617356,0.308027043393035,58.7205574657366));
#41081=CARTESIAN_POINT('Ctrl Pts',(1.19882200432129,0.117592859530876,58.7126323439708));
#41082=CARTESIAN_POINT('Ctrl Pts',(1.20151341066637,-0.085835905345154,
58.7047072222051));
#41083=CARTESIAN_POINT('Ctrl Pts',(1.15546001023758,-0.277555573681085,
58.6967821004394));
#41084=CARTESIAN_POINT('Ctrl Pts',(1.10940660980879,-0.469275242017015,
58.6888569786737));
#41085=CARTESIAN_POINT('Ctrl Pts',(1.01460840260613,-0.649285813812847,
58.680931856908));
#41086=CARTESIAN_POINT('Ctrl Pts',(0.88257735128077,-0.795727434958663,
58.6730067351423));
#41087=CARTESIAN_POINT('Ctrl Pts',(0.750546299955413,-0.942169056104479,
58.6650816133765));
#41088=CARTESIAN_POINT('Ctrl Pts',(0.581282404507365,-1.05504172660028,
58.6571564916108));
#41089=CARTESIAN_POINT('Ctrl Pts',(0.395340480265844,-1.12063858420226,
58.6492313698451));
#41090=CARTESIAN_POINT('Ctrl Pts',(0.209398556024328,-1.18623544180424,
58.6413062480794));
#41091=CARTESIAN_POINT('Ctrl Pts',(0.00677860298933977,-1.20455648651239,
58.6333811263137));
#41092=CARTESIAN_POINT('Ctrl Pts',(-0.187913920565669,-1.17337687474967,
58.625456004548));
#41093=CARTESIAN_POINT('Ctrl Pts',(-0.382606444120684,-1.14219726298696,
58.6175308827822));
#41094=CARTESIAN_POINT('Ctrl Pts',(-0.569371538195719,-1.06151699475336,
58.6096057610165));
#41095=CARTESIAN_POINT('Ctrl Pts',(-0.725529103124543,-0.941133599580297,
58.6016806392508));
#41096=CARTESIAN_POINT('Ctrl Pts',(-0.881686668053367,-0.820750204407234,
58.5937555174851));
#41097=CARTESIAN_POINT('Ctrl Pts',(-1.00723670383598,-0.660663682294702,
58.5858303957194));
#41098=CARTESIAN_POINT('Ctrl Pts',(-1.08693285333723,-0.480314380459157,
58.5779052739537));
#41099=CARTESIAN_POINT('Ctrl Pts',(-1.15352848109623,-0.329611052295889,
58.5712828905342));
#41100=CARTESIAN_POINT('Ctrl Pts',(-1.18810620429966,-0.164759048855221,
58.5646605071147));
#41101=CARTESIAN_POINT('Ctrl Pts',(-1.18826810796675,2.71338473248756E-5,
58.5580381236952));
#41102=CARTESIAN_POINT('Ctrl Pts',(-1.18824324986219,2.98497152091627E-5,
58.5155118763048));
#41103=CARTESIAN_POINT('Ctrl Pts',(-1.18808231114118,-0.156753103451461,
58.5218122478379));
#41104=CARTESIAN_POINT('Ctrl Pts',(-1.15687154130276,-0.313598226513166,
58.528112619371));
#41105=CARTESIAN_POINT('Ctrl Pts',(-1.09642773814146,-0.458226093307908,
58.534412990904));
#41106=CARTESIAN_POINT('Ctrl Pts',(-1.02039658703845,-0.640150833626332,
58.5423381126698));
#41107=CARTESIAN_POINT('Ctrl Pts',(-0.898110993753373,-0.802744621614826,
58.5502632344355));
#41108=CARTESIAN_POINT('Ctrl Pts',(-0.744420892944448,-0.926262636460101,
58.5581883562012));
#41109=CARTESIAN_POINT('Ctrl Pts',(-0.590730792135523,-1.04978065130538,
58.5661134779669));
#41110=CARTESIAN_POINT('Ctrl Pts',(-0.405636183802751,-1.13422289300743,
58.5740385997326));
#41111=CARTESIAN_POINT('Ctrl Pts',(-0.211614309667662,-1.16933499113732,
58.5819637214984));
#41112=CARTESIAN_POINT('Ctrl Pts',(-0.0175924355325727,-1.2044470892672,
58.5898888432641));
#41113=CARTESIAN_POINT('Ctrl Pts',(0.185356704404831,-1.19022904382492,
58.5978139650298));
#41114=CARTESIAN_POINT('Ctrl Pts',(0.372587676565259,-1.12840744451015,
58.6057390867955));
#41115=CARTESIAN_POINT('Ctrl Pts',(0.559818648725685,-1.06658584519538,
58.6136642085613));
#41116=CARTESIAN_POINT('Ctrl Pts',(0.731331453109135,-0.95716069200813,
58.6215893303269));
#41117=CARTESIAN_POINT('Ctrl Pts',(0.866298174752611,-0.813420192750661,
58.6295144520927));
#41118=CARTESIAN_POINT('Ctrl Pts',(1.00126489639609,-0.669679693493192,
58.6374395738584));
#41119=CARTESIAN_POINT('Ctrl Pts',(1.09968553529959,-0.491623848165508,
58.6453646956241));
#41120=CARTESIAN_POINT('Ctrl Pts',(1.14960823337849,-0.300875135733428,
58.6532898173898));
#41121=CARTESIAN_POINT('Ctrl Pts',(1.1995309314574,-0.110126423301345,58.6612149391555));
#41122=CARTESIAN_POINT('Ctrl Pts',(1.20095568871171,0.0933151562351321,
58.6691400609212));
#41123=CARTESIAN_POINT('Ctrl Pts',(1.15370948760467,0.284744369154499,58.677065182687));
#41124=CARTESIAN_POINT('Ctrl Pts',(1.10646328649763,0.476173582073863,58.6849903044527));
#41125=CARTESIAN_POINT('Ctrl Pts',(1.01054612702925,0.655590428376123,58.6929154262184));
#41126=CARTESIAN_POINT('Ctrl Pts',(0.877605853499431,0.801207153898268,
58.7008405479841));
#41127=CARTESIAN_POINT('Ctrl Pts',(0.744665579969613,0.946823879420414,
58.7087656697499));
#41128=CARTESIAN_POINT('Ctrl Pts',(0.574702192378362,1.05864048416245,58.7166907915156));
#41129=CARTESIAN_POINT('Ctrl Pts',(0.38835544993374,1.12307835081128,58.7246159132813));
#41130=CARTESIAN_POINT('Ctrl Pts',(0.202008707489123,1.18751621746011,58.732541035047));
#41131=CARTESIAN_POINT('Ctrl Pts',(-0.000721389808862383,1.20457534601574,
58.7404661568127));
#41132=CARTESIAN_POINT('Ctrl Pts',(-0.195216008152784,1.17218413558413,
58.7483912785784));
#41133=CARTESIAN_POINT('Ctrl Pts',(-0.389710626496712,1.13979292515252,
58.7563164003441));
#41134=CARTESIAN_POINT('Ctrl Pts',(-0.575969765886575,1.05795137573367,
58.7642415221098));
#41135=CARTESIAN_POINT('Ctrl Pts',(-0.731374768023134,0.936598038783625,
58.7721666438756));
#41136=CARTESIAN_POINT('Ctrl Pts',(-0.886779770159693,0.815244701833581,
58.7800917656413));
#41137=CARTESIAN_POINT('Ctrl Pts',(-1.01133063504295,0.654379577352344,
58.788016887407));
#41138=CARTESIAN_POINT('Ctrl Pts',(-1.08990234135637,0.473537563304248,
58.7959420091728));
#41139=CARTESIAN_POINT('Ctrl Pts',(-1.15457591560756,0.324683733191172,
58.8024652982168));
#41140=CARTESIAN_POINT('Ctrl Pts',(-1.18809774503898,0.16229518462225,58.8089885872608));
#41141=CARTESIAN_POINT('Ctrl Pts',(-1.1882605894663,-2.81773776290431E-5,
58.8155118763048));
#41142=CARTESIAN_POINT('Origin',(0.,0.,57.95));
#41143=CARTESIAN_POINT('',(-1.18814215656827,1.71474778534464E-5,59.1580381236952));
#41144=CARTESIAN_POINT('',(-1.18813194074363,1.05284942013778E-5,59.1155118763048));
#41145=CARTESIAN_POINT('',(-1.188225,-1.45515594291686E-16,57.95));
#41146=CARTESIAN_POINT('Ctrl Pts',(-1.18814215656827,1.71474778534464E-5,
59.1580381236952));
#41147=CARTESIAN_POINT('Ctrl Pts',(-1.18818264834069,0.0790378129302419,
59.1548634294919));
#41148=CARTESIAN_POINT('Ctrl Pts',(-1.18041668547805,0.15805062590395,59.1516887352886));
#41149=CARTESIAN_POINT('Ctrl Pts',(-1.16476568243126,0.235469396674217,
59.1485140410854));
#41150=CARTESIAN_POINT('Ctrl Pts',(-1.12569542968893,0.428733108396165,
59.1405889193196));
#41151=CARTESIAN_POINT('Ctrl Pts',(-1.03748779648867,0.61206319183124,59.1326637975539));
#41152=CARTESIAN_POINT('Ctrl Pts',(-0.910854409230566,0.763196682988669,
59.1247386757882));
#41153=CARTESIAN_POINT('Ctrl Pts',(-0.78422102197246,0.914330174146098,
59.1168135540225));
#41154=CARTESIAN_POINT('Ctrl Pts',(-0.619161880656503,1.03326707302588,
59.1088884322568));
#41155=CARTESIAN_POINT('Ctrl Pts',(-0.43572118997955,1.10556409870368,59.100963310491));
#41156=CARTESIAN_POINT('Ctrl Pts',(-0.252280499302597,1.17786112438148,
59.0930381887253));
#41157=CARTESIAN_POINT('Ctrl Pts',(-0.0504582592646509,1.20351827685729,
59.0851130669596));
#41158=CARTESIAN_POINT('Ctrl Pts',(0.145236943336567,1.17941984129059,59.0771879451939));
#41159=CARTESIAN_POINT('Ctrl Pts',(0.340932145937779,1.15532140572389,59.0692628234282));
#41160=CARTESIAN_POINT('Ctrl Pts',(0.53050031110226,1.08146738211468,59.0613377016625));
#41161=CARTESIAN_POINT('Ctrl Pts',(0.690920944016633,0.966826344727343,
59.0534125798967));
#41162=CARTESIAN_POINT('Ctrl Pts',(0.851341576931016,0.852185307340005,
59.045487458131));
#41163=CARTESIAN_POINT('Ctrl Pts',(0.982614677595285,0.696757256174546,
59.0375623363653));
#41164=CARTESIAN_POINT('Ctrl Pts',(1.06879889989599,0.519416830032286,59.0296372145996));
#41165=CARTESIAN_POINT('Ctrl Pts',(1.1549831221967,0.342076403890031,59.0217120928339));
#41166=CARTESIAN_POINT('Ctrl Pts',(1.19607846613384,0.142823602770977,59.0137869710682));
#41167=CARTESIAN_POINT('Ctrl Pts',(1.18709445690308,-0.0541450102008245,
59.0058618493024));
#41168=CARTESIAN_POINT('Ctrl Pts',(1.17811044767232,-0.251113623172624,
58.9979367275367));
#41169=CARTESIAN_POINT('Ctrl Pts',(1.11904708527366,-0.445798047997178,
58.990011605771));
#41170=CARTESIAN_POINT('Ctrl Pts',(1.01707681781609,-0.614556489186126,
58.9820864840053));
#41171=CARTESIAN_POINT('Ctrl Pts',(0.915106550358513,-0.783314930375073,
58.9741613622396));
#41172=CARTESIAN_POINT('Ctrl Pts',(0.770229377842034,-0.926147387928421,
58.9662362404738));
#41173=CARTESIAN_POINT('Ctrl Pts',(0.600038677274853,-1.02570878787008,
58.9583111187081));
#41174=CARTESIAN_POINT('Ctrl Pts',(0.429847976707667,-1.12527018781175,
58.9503859969424));
#41175=CARTESIAN_POINT('Ctrl Pts',(0.234343748089779,-1.18156053014173,
58.9424608751767));
#41176=CARTESIAN_POINT('Ctrl Pts',(0.0372673410142875,-1.18774411260734,
58.934535753411));
#41177=CARTESIAN_POINT('Ctrl Pts',(-0.159809066061204,-1.19392769507295,
58.9266106316453));
#41178=CARTESIAN_POINT('Ctrl Pts',(-0.358457651594298,-1.1500045176742,
58.9186855098796));
#41179=CARTESIAN_POINT('Ctrl Pts',(-0.534555226287983,-1.06130845741842,
58.9107603881138));
#41180=CARTESIAN_POINT('Ctrl Pts',(-0.710652800981668,-0.97261239716265,
58.9028352663481));
#41181=CARTESIAN_POINT('Ctrl Pts',(-0.864199364835943,-0.839143454049854,
58.8949101445824));
#41182=CARTESIAN_POINT('Ctrl Pts',(-0.976548760286572,-0.677109629618743,
58.8869850228167));
#41183=CARTESIAN_POINT('Ctrl Pts',(-1.0888981557372,-0.515075805187633,
58.8790599010509));
#41184=CARTESIAN_POINT('Ctrl Pts',(-1.16005038278419,-0.324477099438208,
58.8711347792852));
#41185=CARTESIAN_POINT('Ctrl Pts',(-1.18136496388598,-0.128459152427356,
58.8632096575195));
#41186=CARTESIAN_POINT('Ctrl Pts',(-1.18600123658848,-0.085822018130073,
58.8614858129114));
#41187=CARTESIAN_POINT('Ctrl Pts',(-1.18827951981344,-0.0429284809945659,
58.8597619683033));
#41188=CARTESIAN_POINT('Ctrl Pts',(-1.18823546047583,-3.02886631483035E-5,
58.8580381236952));
#41189=CARTESIAN_POINT('Ctrl Pts',(-1.1882605894663,-2.81773776290431E-5,
58.8155118763048));
#41190=CARTESIAN_POINT('Ctrl Pts',(-1.1882955841822,-0.0349109180948725,
58.8169137090265));
#41191=CARTESIAN_POINT('Ctrl Pts',(-1.1867900424793,-0.069790648460224,
58.8183155417482));
#41192=CARTESIAN_POINT('Ctrl Pts',(-1.18372205960733,-0.10453240240814,
58.8197173744699));
#41193=CARTESIAN_POINT('Ctrl Pts',(-1.16637752380126,-0.300941450457477,
58.8276424962356));
#41194=CARTESIAN_POINT('Ctrl Pts',(-1.09909590444552,-0.492940642941198,
58.8355676180013));
#41195=CARTESIAN_POINT('Ctrl Pts',(-0.990047646024145,-0.657214269592707,
58.843492739767));
#41196=CARTESIAN_POINT('Ctrl Pts',(-0.880999387602772,-0.821487896244211,
58.8514178615328));
#41197=CARTESIAN_POINT('Ctrl Pts',(-0.730184490115758,-0.958035957063507,
58.8593429832985));
#41198=CARTESIAN_POINT('Ctrl Pts',(-0.555917387119857,-1.05027653322925,
58.8672681050642));
#41199=CARTESIAN_POINT('Ctrl Pts',(-0.381650284123952,-1.142517109395,58.8751932268299));
#41200=CARTESIAN_POINT('Ctrl Pts',(-0.183930975619157,-1.1904502009072,
58.8831183485956));
#41201=CARTESIAN_POINT('Ctrl Pts',(0.0132301972489506,-1.1882549808164,
58.8910434703614));
#41202=CARTESIAN_POINT('Ctrl Pts',(0.210391370117058,-1.1860597607256,58.8989685921271));
#41203=CARTESIAN_POINT('Ctrl Pts',(0.406994407348479,-1.13373622903181,
58.9068937138928));
#41204=CARTESIAN_POINT('Ctrl Pts',(0.579164523876036,-1.03763837238109,
58.9148188356585));
#41205=CARTESIAN_POINT('Ctrl Pts',(0.751334640403598,-0.941540515730364,
58.9227439574242));
#41206=CARTESIAN_POINT('Ctrl Pts',(0.899071836227295,-0.801668334122712,
58.93066907919));
#41207=CARTESIAN_POINT('Ctrl Pts',(1.00443542311368,-0.635007415979277,
58.9385942009557));
#41208=CARTESIAN_POINT('Ctrl Pts',(1.10979901000005,-0.468346497835848,
58.9465193227214));
#41209=CARTESIAN_POINT('Ctrl Pts',(1.17278898794912,-0.274896843156645,
58.9544444444871));
#41210=CARTESIAN_POINT('Ctrl Pts',(1.18575607439587,-0.0781503012631315,
58.9623695662528));
#41211=CARTESIAN_POINT('Ctrl Pts',(1.19872316084263,0.11859624063038,58.9702946880185));
#41212=CARTESIAN_POINT('Ctrl Pts',(1.16166735578707,0.318639669738194,58.9782198097842));
#41213=CARTESIAN_POINT('Ctrl Pts',(1.07908858656325,0.497687411839151,58.98614493155));
#41214=CARTESIAN_POINT('Ctrl Pts',(0.996509817339424,0.676735153940114,
58.9940700533157));
#41215=CARTESIAN_POINT('Ctrl Pts',(0.868408083947323,0.834787209034219,
59.0019951750814));
#41216=CARTESIAN_POINT('Ctrl Pts',(0.710339612753224,0.952650288462575,
59.0099202968471));
#41217=CARTESIAN_POINT('Ctrl Pts',(0.552271141559124,1.07051336789093,59.0178454186129));
#41218=CARTESIAN_POINT('Ctrl Pts',(0.364235932563025,1.14818747165354,59.0257705403786));
#41219=CARTESIAN_POINT('Ctrl Pts',(0.169068323743945,1.17624012831591,59.0336956621443));
#41220=CARTESIAN_POINT('Ctrl Pts',(-0.0260992850751359,1.20429278497829,
59.04162078391));
#41221=CARTESIAN_POINT('Ctrl Pts',(-0.228399293717199,1.18272399454044,
59.0495459056757));
#41222=CARTESIAN_POINT('Ctrl Pts',(-0.41326509683661,1.11415299545927,59.0574710274414));
#41223=CARTESIAN_POINT('Ctrl Pts',(-0.598130899956021,1.04558199637809,
59.0653961492071));
#41224=CARTESIAN_POINT('Ctrl Pts',(-0.765562497552781,0.930008788653607,
59.0733212709729));
#41225=CARTESIAN_POINT('Ctrl Pts',(-0.895227582138825,0.781468178323405,
59.0812463927386));
#41226=CARTESIAN_POINT('Ctrl Pts',(-1.02489266672487,0.632927567993202,
59.0891715145043));
#41227=CARTESIAN_POINT('Ctrl Pts',(-1.1167912383002,0.451419555057285,59.09709663627));
#41228=CARTESIAN_POINT('Ctrl Pts',(-1.15976345582045,0.258985837639138,
59.1050217580358));
#41229=CARTESIAN_POINT('Ctrl Pts',(-1.17872357014204,0.174080624640588,
59.1085184641254));
#41230=CARTESIAN_POINT('Ctrl Pts',(-1.18815903006735,0.0870484687860079,
59.1120151702151));
#41231=CARTESIAN_POINT('Ctrl Pts',(-1.18813194074363,1.05284942013778E-5,
59.1155118763048));
#41232=CARTESIAN_POINT('Origin',(0.,0.,57.95));
#41233=CARTESIAN_POINT('',(-1.18832756091501,3.87725375256866E-6,59.4580381236952));
#41234=CARTESIAN_POINT('',(-1.18831870923562,1.19544632238963E-5,59.4155118763048));
#41235=CARTESIAN_POINT('',(-1.188225,-1.45515594291686E-16,57.95));
#41236=CARTESIAN_POINT('Ctrl Pts',(-1.18832756091501,3.87725375256866E-6,
59.4580381236952));
#41237=CARTESIAN_POINT('Ctrl Pts',(-1.18832824821205,0.00368882683057432,
59.4578900124462));
#41238=CARTESIAN_POINT('Ctrl Pts',(-1.18831146503093,0.00737377012193548,
59.4577419011973));
#41239=CARTESIAN_POINT('Ctrl Pts',(-1.18827717308989,0.0110585504702445,
59.4575937899484));
#41240=CARTESIAN_POINT('Ctrl Pts',(-1.18644228336852,0.208223405601848,
59.4496686681827));
#41241=CARTESIAN_POINT('Ctrl Pts',(-1.13447814598937,0.404921739252035,
59.4417435464169));
#41242=CARTESIAN_POINT('Ctrl Pts',(-1.03869510378624,0.577267193901848,
59.4338184246512));
#41243=CARTESIAN_POINT('Ctrl Pts',(-0.942912061583119,0.749612648551651,
59.4258933028855));
#41244=CARTESIAN_POINT('Ctrl Pts',(-0.803310114556024,0.897605224201085,
59.4179681811198));
#41245=CARTESIAN_POINT('Ctrl Pts',(-0.636842034887918,1.00327322017851,
59.4100430593541));
#41246=CARTESIAN_POINT('Ctrl Pts',(-0.470373955219807,1.10894121615594,
59.4021179375883));
#41247=CARTESIAN_POINT('Ctrl Pts',(-0.277039742910682,1.17228463246137,
59.3941928158226));
#41248=CARTESIAN_POINT('Ctrl Pts',(-0.0803172283162318,1.18561126621479,
59.3862676940569));
#41249=CARTESIAN_POINT('Ctrl Pts',(0.116405286278219,1.19893789996821,59.3783425722912));
#41250=CARTESIAN_POINT('Ctrl Pts',(0.316516103157997,1.16224775116963,59.3704174505255));
#41251=CARTESIAN_POINT('Ctrl Pts',(0.49571446474428,1.07999634313522,59.3624923287597));
#41252=CARTESIAN_POINT('Ctrl Pts',(0.674912826330568,0.997744935100801,
59.354567206994));
#41253=CARTESIAN_POINT('Ctrl Pts',(0.833198732623362,0.869932267830549,
59.3466420852283));
#41254=CARTESIAN_POINT('Ctrl Pts',(0.951350496902659,0.712079464512692,
59.3387169634626));
#41255=CARTESIAN_POINT('Ctrl Pts',(1.06950226118195,0.554226661194839,59.3307918416969));
#41256=CARTESIAN_POINT('Ctrl Pts',(1.14751988344775,0.366333721829396,59.3228667199312));
#41257=CARTESIAN_POINT('Ctrl Pts',(1.17592917657546,0.171217707668849,59.3149415981654));
#41258=CARTESIAN_POINT('Ctrl Pts',(1.20433846970317,-0.0238983064916926,
59.3070164763997));
#41259=CARTESIAN_POINT('Ctrl Pts',(1.18313943369279,-0.226237395447325,
59.299091354634));
#41260=CARTESIAN_POINT('Ctrl Pts',(1.1149064053193,-0.411228208075728,59.2911662328683));
#41261=CARTESIAN_POINT('Ctrl Pts',(1.04667337694581,-0.596219020704137,
59.2832411111026));
#41262=CARTESIAN_POINT('Ctrl Pts',(0.931406356209218,-0.76386155700532,
59.2753159893369));
#41263=CARTESIAN_POINT('Ctrl Pts',(0.783102966869399,-0.893797893832923,
59.2673908675711));
#41264=CARTESIAN_POINT('Ctrl Pts',(0.634799577529581,-1.02373423066053,
59.2594657458054));
#41265=CARTESIAN_POINT('Ctrl Pts',(0.453459819586538,-1.11596436801455,
59.2515406240397));
#41266=CARTESIAN_POINT('Ctrl Pts',(0.26110495886651,-1.15928820066236,59.243615502274));
#41267=CARTESIAN_POINT('Ctrl Pts',(0.0687500981464874,-1.20261203331017,
59.2356903805083));
#41268=CARTESIAN_POINT('Ctrl Pts',(-0.134619865350523,-1.19702956125176,
59.2277652587426));
#41269=CARTESIAN_POINT('Ctrl Pts',(-0.324308394704534,-1.14321870036482,
59.2198401369768));
#41270=CARTESIAN_POINT('Ctrl Pts',(-0.513996924058551,-1.08940783947788,
59.2119150152111));
#41271=CARTESIAN_POINT('Ctrl Pts',(-0.690004019269572,-0.987368589762404,
59.2039898934454));
#41272=CARTESIAN_POINT('Ctrl Pts',(-0.830955994418717,-0.849492240741074,
59.1960647716797));
#41273=CARTESIAN_POINT('Ctrl Pts',(-0.971907969567863,-0.711615891719744,
59.1881396499139));
#41274=CARTESIAN_POINT('Ctrl Pts',(-1.07780482465514,-0.537902443392555,
59.1802145281482));
#41275=CARTESIAN_POINT('Ctrl Pts',(-1.13578681605657,-0.349447049224552,
59.1722894063825));
#41276=CARTESIAN_POINT('Ctrl Pts',(-1.17054202338604,-0.236484280296531,
59.1675389788201));
#41277=CARTESIAN_POINT('Ctrl Pts',(-1.18808156703762,-0.118224775407469,
59.1627885512576));
#41278=CARTESIAN_POINT('Ctrl Pts',(-1.18814215656827,1.71474778534464E-5,
59.1580381236952));
#41279=CARTESIAN_POINT('Ctrl Pts',(-1.18813194074363,1.05284942013778E-5,
59.1155118763048));
#41280=CARTESIAN_POINT('Ctrl Pts',(-1.18809763337471,-0.110218975876756,
59.1199402919808));
#41281=CARTESIAN_POINT('Ctrl Pts',(-1.17288630091938,-0.220457757932465,
59.1243687076569));
#41282=CARTESIAN_POINT('Ctrl Pts',(-1.14262409572745,-0.326397171276419,
59.1287971233329));
#41283=CARTESIAN_POINT('Ctrl Pts',(-1.08846665464904,-0.51598704087343,
59.1367222450986));
#41284=CARTESIAN_POINT('Ctrl Pts',(-0.986105909027061,-0.691807358167079,
59.1446473668643));
#41285=CARTESIAN_POINT('Ctrl Pts',(-0.847972189722383,-0.83250711889548,
59.1525724886301));
#41286=CARTESIAN_POINT('Ctrl Pts',(-0.709838470417701,-0.973206879623886,
59.1604976103958));
#41287=CARTESIAN_POINT('Ctrl Pts',(-0.535931777430326,-1.07878608378704,
59.1684227321615));
#41288=CARTESIAN_POINT('Ctrl Pts',(-0.347370731180798,-1.13642356217792,
59.1763478539272));
#41289=CARTESIAN_POINT('Ctrl Pts',(-0.158809684931281,-1.19406104056879,
59.1842729756929));
#41290=CARTESIAN_POINT('Ctrl Pts',(0.0444057145803972,-1.2037567931874,
59.1921980974586));
#41291=CARTESIAN_POINT('Ctrl Pts',(0.237597700143673,-1.16433340175427,
59.2001232192244));
#41292=CARTESIAN_POINT('Ctrl Pts',(0.430789685706959,-1.12491001032114,
59.2080483409901));
#41293=CARTESIAN_POINT('Ctrl Pts',(0.613958257321854,-1.03636747483627,
59.2159734627558));
#41294=CARTESIAN_POINT('Ctrl Pts',(0.764860064428019,-0.909458091061591,
59.2238985845215));
#41295=CARTESIAN_POINT('Ctrl Pts',(0.915761871534184,-0.782548707286909,
59.2318237062872));
#41296=CARTESIAN_POINT('Ctrl Pts',(1.03439691413161,-0.617272475222414,
59.239748828053));
#41297=CARTESIAN_POINT('Ctrl Pts',(1.10635856766692,-0.433699962306019,
59.2476739498187));
#41298=CARTESIAN_POINT('Ctrl Pts',(1.17832022120222,-0.250127449389618,
59.2555990715844));
#41299=CARTESIAN_POINT('Ctrl Pts',(1.20360848567539,-0.0482586556213197,
59.2635241933501));
#41300=CARTESIAN_POINT('Ctrl Pts',(1.17915244271448,0.147392178878999,59.2714493151158));
#41301=CARTESIAN_POINT('Ctrl Pts',(1.15469639975357,0.343043013379306,59.2793744368816));
#41302=CARTESIAN_POINT('Ctrl Pts',(1.08049604935858,0.532475888611629,59.2872995586473));
#41303=CARTESIAN_POINT('Ctrl Pts',(0.965562022507184,0.692686738898676,
59.295224680413));
#41304=CARTESIAN_POINT('Ctrl Pts',(0.850627995655786,0.852897589185722,
59.3031498021787));
#41305=CARTESIAN_POINT('Ctrl Pts',(0.694960292347977,0.983886414527489,
59.3110749239444));
#41306=CARTESIAN_POINT('Ctrl Pts',(0.51746265390297,1.06974639021121,59.3190000457101));
#41307=CARTESIAN_POINT('Ctrl Pts',(0.339965015457963,1.15560636589492,59.3269251674758));
#41308=CARTESIAN_POINT('Ctrl Pts',(0.140637441875762,1.19633749192059,59.3348502892416));
#41309=CARTESIAN_POINT('Ctrl Pts',(-0.0563144236134591,1.18699352283291,
59.3427754110073));
#41310=CARTESIAN_POINT('Ctrl Pts',(-0.253266289102692,1.17764955374524,
59.350700532773));
#41311=CARTESIAN_POINT('Ctrl Pts',(-0.447842446498957,1.11823048954422,
59.3586256545387));
#41312=CARTESIAN_POINT('Ctrl Pts',(-0.616414247931142,1.01595197352132,
59.3665507763045));
#41313=CARTESIAN_POINT('Ctrl Pts',(-0.784986049363317,0.913673457498427,
59.3744758980702));
#41314=CARTESIAN_POINT('Ctrl Pts',(-0.927553494831426,0.768535489653664,
59.3824010198359));
#41315=CARTESIAN_POINT('Ctrl Pts',(-1.02680369250096,0.598163117067689,
59.3903261416016));
#41316=CARTESIAN_POINT('Ctrl Pts',(-1.12605389017049,0.427790744481714,
59.3982512633673));
#41317=CARTESIAN_POINT('Ctrl Pts',(-1.18198684004144,0.23218396715453,59.406176385133));
#41318=CARTESIAN_POINT('Ctrl Pts',(-1.18781024034888,0.0350965878354738,
59.4141015068987));
#41319=CARTESIAN_POINT('Ctrl Pts',(-1.18815568806463,0.0234052423339456,
59.4145716300341));
#41320=CARTESIAN_POINT('Ctrl Pts',(-1.18832480348564,0.0117086866888603,
59.4150417531695));
#41321=CARTESIAN_POINT('Ctrl Pts',(-1.18831870923562,1.19544632238963E-5,
59.4155118763048));
#41322=CARTESIAN_POINT('Origin',(0.,0.,57.95));
#41323=CARTESIAN_POINT('',(-1.18815715028295,-2.22996587661006E-5,59.7580381236952));
#41324=CARTESIAN_POINT('',(-1.1881744462934,-2.6792430042513E-5,59.7155118763048));
#41325=CARTESIAN_POINT('',(-1.188225,-1.45515594291686E-16,57.95));
#41326=CARTESIAN_POINT('Ctrl Pts',(-1.18815715028295,-2.22996587661006E-5,
59.7580381236952));
#41327=CARTESIAN_POINT('Ctrl Pts',(-1.18807148486871,0.125588696935144,
59.7529914736348));
#41328=CARTESIAN_POINT('Ctrl Pts',(-1.16823594397195,0.25122604577743,59.7479448235745));
#41329=CARTESIAN_POINT('Ctrl Pts',(-1.12908604691359,0.370524885226803,
59.7428981735142));
#41330=CARTESIAN_POINT('Ctrl Pts',(-1.06760611515802,0.557868532566024,
59.7349730517485));
#41331=CARTESIAN_POINT('Ctrl Pts',(-0.958495617630607,0.729580968281685,
59.7270479299828));
#41332=CARTESIAN_POINT('Ctrl Pts',(-0.815002291341349,0.864810140128416,
59.7191228082171));
#41333=CARTESIAN_POINT('Ctrl Pts',(-0.671508965052082,1.00003931197515,
59.7111976864513));
#41334=CARTESIAN_POINT('Ctrl Pts',(-0.493632810000966,1.09878521995296,
59.7032725646856));
#41335=CARTESIAN_POINT('Ctrl Pts',(-0.302975525170295,1.14905644757922,
59.6953474429199));
#41336=CARTESIAN_POINT('Ctrl Pts',(-0.11231824033963,1.19932767520548,59.6874223211542));
#41337=CARTESIAN_POINT('Ctrl Pts',(0.0911201742705878,1.2011242224802,59.6794971993885));
#41338=CARTESIAN_POINT('Ctrl Pts',(0.282635353985177,1.15422794809806,59.6715720776228));
#41339=CARTESIAN_POINT('Ctrl Pts',(0.474150533699762,1.10733167371592,59.663646955857));
#41340=CARTESIAN_POINT('Ctrl Pts',(0.653742478518715,1.01174257767693,59.6557218340913));
#41341=CARTESIAN_POINT('Ctrl Pts',(0.799601946393605,0.879068653271273,
59.6477967123256));
#41342=CARTESIAN_POINT('Ctrl Pts',(0.9454614142685,0.746394728865611,59.6398715905599));
#41343=CARTESIAN_POINT('Ctrl Pts',(1.05758840519933,0.576635976093282,59.6319464687942));
#41344=CARTESIAN_POINT('Ctrl Pts',(1.12236671392606,0.390407309550219,59.6240213470285));
#41345=CARTESIAN_POINT('Ctrl Pts',(1.18714502265279,0.204178643007155,59.6160962252628));
#41346=CARTESIAN_POINT('Ctrl Pts',(1.20457464917542,0.0014800626933443,
59.608171103497));
#41347=CARTESIAN_POINT('Ctrl Pts',(1.17253895226116,-0.193073427482673,
59.6002459817313));
#41348=CARTESIAN_POINT('Ctrl Pts',(1.1405032553469,-0.387626917658684,59.5923208599656));
#41349=CARTESIAN_POINT('Ctrl Pts',(1.05900223499575,-0.574035317696915,
59.5843957381999));
#41350=CARTESIAN_POINT('Ctrl Pts',(0.937933112448952,-0.729661842412061,
59.5764706164341));
#41351=CARTESIAN_POINT('Ctrl Pts',(0.816863989902144,-0.885288367127217,
59.5685454946684));
#41352=CARTESIAN_POINT('Ctrl Pts',(0.656226765159698,-1.01013301651927,
59.5606203729027));
#41353=CARTESIAN_POINT('Ctrl Pts',(0.47552865042574,-1.08903509366436,59.552695251137));
#41354=CARTESIAN_POINT('Ctrl Pts',(0.294830535691792,-1.16793717080945,
59.5447701293713));
#41355=CARTESIAN_POINT('Ctrl Pts',(0.0940715309663313,-1.20089667570757,
59.5368450076055));
#41356=CARTESIAN_POINT('Ctrl Pts',(-0.102368887697813,-1.18391112112818,
59.5289198858398));
#41357=CARTESIAN_POINT('Ctrl Pts',(-0.298809306361958,-1.16692556654879,
59.5209947640741));
#41358=CARTESIAN_POINT('Ctrl Pts',(-0.4909311389648,-1.09999495249189,59.5130696423084));
#41359=CARTESIAN_POINT('Ctrl Pts',(-0.655403784494695,-0.991247098705512,
59.5051445205427));
#41360=CARTESIAN_POINT('Ctrl Pts',(-0.819876430024596,-0.882499244919128,
59.497219398777));
#41361=CARTESIAN_POINT('Ctrl Pts',(-0.956699888481545,-0.731934151403257,
59.4892942770112));
#41362=CARTESIAN_POINT('Ctrl Pts',(-1.04925879667821,-0.557835916338813,
59.4813691552455));
#41363=CARTESIAN_POINT('Ctrl Pts',(-1.14008788722682,-0.38699137349458,
59.4735921447287));
#41364=CARTESIAN_POINT('Ctrl Pts',(-1.18829147239159,-0.193485083363211,
59.465815134212));
#41365=CARTESIAN_POINT('Ctrl Pts',(-1.18832756091501,3.87725375256866E-6,
59.4580381236952));
#41366=CARTESIAN_POINT('Ctrl Pts',(-1.18831870923562,1.19544632238963E-5,
59.4155118763048));
#41367=CARTESIAN_POINT('Ctrl Pts',(-1.18822206939351,-0.185469499572606,
59.4229668749352));
#41368=CARTESIAN_POINT('Ctrl Pts',(-1.14406690366381,-0.370995356858145,
59.4304218735655));
#41369=CARTESIAN_POINT('Ctrl Pts',(-1.06032974762535,-0.536493955094488,
59.4378768721959));
#41370=CARTESIAN_POINT('Ctrl Pts',(-0.97131200385046,-0.712429137394463,
59.4458019939616));
#41371=CARTESIAN_POINT('Ctrl Pts',(-0.837562665556747,-0.865731520683477,
59.4537271157273));
#41372=CARTESIAN_POINT('Ctrl Pts',(-0.67532378448248,-0.977784599832173,
59.4616522374931));
#41373=CARTESIAN_POINT('Ctrl Pts',(-0.513084903408217,-1.08983767898087,
59.4695773592588));
#41374=CARTESIAN_POINT('Ctrl Pts',(-0.322356479553399,-1.16064145398924,
59.4775024810245));
#41375=CARTESIAN_POINT('Ctrl Pts',(-0.126299905510072,-1.18159776210965,
59.4854276027902));
#41376=CARTESIAN_POINT('Ctrl Pts',(0.0697566685332563,-1.20255407023006,
59.4933527245559));
#41377=CARTESIAN_POINT('Ctrl Pts',(0.271141392765097,-1.17366291146249,
59.5012778463217));
#41378=CARTESIAN_POINT('Ctrl Pts',(0.453398810824565,-1.09843272706388,
59.5092029680874));
#41379=CARTESIAN_POINT('Ctrl Pts',(0.635656228884028,-1.02320254266526,
59.5171280898531));
#41380=CARTESIAN_POINT('Ctrl Pts',(0.798786340771123,-0.901633332635603,
59.5250532116188));
#41381=CARTESIAN_POINT('Ctrl Pts',(0.922979196271283,-0.748488036544175,
59.5329783333845));
#41382=CARTESIAN_POINT('Ctrl Pts',(1.04717205177145,-0.595342740452742,
59.5409034551503));
#41383=CARTESIAN_POINT('Ctrl Pts',(1.13242765088467,-0.410621358299555,
59.548828576916));
#41384=CARTESIAN_POINT('Ctrl Pts',(1.16839285212588,-0.216755808551492,
59.5567536986817));
#41385=CARTESIAN_POINT('Ctrl Pts',(1.20435805336708,-0.0228902588034223,
59.5646788204474));
#41386=CARTESIAN_POINT('Ctrl Pts',(1.19103285673626,0.180119458539511,59.5726039422131));
#41387=CARTESIAN_POINT('Ctrl Pts',(1.13003542701731,0.367620553647926,59.5805290639788));
#41388=CARTESIAN_POINT('Ctrl Pts',(1.06903799729836,0.555121648756329,59.5884541857445));
#41389=CARTESIAN_POINT('Ctrl Pts',(0.960368334491289,0.72711412163022,59.5963793075103));
#41390=CARTESIAN_POINT('Ctrl Pts',(0.817222903323089,0.862711807917861,
59.604304429276));
#41391=CARTESIAN_POINT('Ctrl Pts',(0.674077472154888,0.998309494205502,
59.6122295510417));
#41392=CARTESIAN_POINT('Ctrl Pts',(0.496456272625558,1.0975123939069,59.6201546728074));
#41393=CARTESIAN_POINT('Ctrl Pts',(0.305928999608111,1.14827365419266,59.6280797945732));
#41394=CARTESIAN_POINT('Ctrl Pts',(0.115401726590658,1.19903491447843,59.6360049163389));
#41395=CARTESIAN_POINT('Ctrl Pts',(-0.0880316199149155,1.20135453534858,
59.6439300381046));
#41396=CARTESIAN_POINT('Ctrl Pts',(-0.279666801176563,1.15495082957736,
59.6518551598703));
#41397=CARTESIAN_POINT('Ctrl Pts',(-0.47130198243821,1.10854712380614,59.659780281636));
#41398=CARTESIAN_POINT('Ctrl Pts',(-0.651138998455935,1.01342009139355,
59.6677054034017));
#41399=CARTESIAN_POINT('Ctrl Pts',(-0.797339081473339,0.881121627627638,
59.6756305251674));
#41400=CARTESIAN_POINT('Ctrl Pts',(-0.943539164490747,0.748823163861718,
59.6835556469331));
#41401=CARTESIAN_POINT('Ctrl Pts',(-1.05610231450784,0.579353268742461,
59.6914807686989));
#41402=CARTESIAN_POINT('Ctrl Pts',(-1.12135923406337,0.393291770773819,
59.6994058904646));
#41403=CARTESIAN_POINT('Ctrl Pts',(-1.16556579026982,0.267249381340982,
59.7047745524113));
#41404=CARTESIAN_POINT('Ctrl Pts',(-1.18806340877614,0.133593067292119,
59.7101432143581));
#41405=CARTESIAN_POINT('Ctrl Pts',(-1.1881744462934,-2.6792430042513E-5,
59.7155118763048));
#41406=CARTESIAN_POINT('Origin',(0.,0.,55.5071980324285));
#41407=CARTESIAN_POINT('',(-1.01641695750709,-1.90763918373965E-5,59.8571980324285));
#41408=CARTESIAN_POINT('',(-1.016475,-7.2179708060976E-14,59.861775));
#41409=CARTESIAN_POINT('',(-1.016475,-7.2179708060976E-14,55.5071980324285));
#41410=CARTESIAN_POINT('',(-1.01180833082817,-0.0972899136175108,59.861775));
#41411=CARTESIAN_POINT('Ctrl Pts',(-1.01641695750709,-1.90763918375067E-5,
59.8571980324285));
#41412=CARTESIAN_POINT('Ctrl Pts',(-1.01643911175058,-0.0325037918279691,
59.8587236882857));
#41413=CARTESIAN_POINT('Ctrl Pts',(-1.01491718827352,-0.0649864470020175,
59.8602493441428));
#41414=CARTESIAN_POINT('Ctrl Pts',(-1.01184089351567,-0.0973166075163148,
59.861775));
#41415=CARTESIAN_POINT('Origin',(0.,0.,59.861775));
#41416=CARTESIAN_POINT('Origin',(0.,0.,55.5071980324285));
#41417=CARTESIAN_POINT('',(-1.01656273641868,3.31682248127331E-6,59.5571980324285));
#41418=CARTESIAN_POINT('',(-1.01643175349457,-2.29197629572075E-5,59.6163519675715));
#41419=CARTESIAN_POINT('',(-1.016475,-7.2179708060976E-14,55.5071980324285));
#41420=CARTESIAN_POINT('Ctrl Pts',(-1.01656273641868,3.31682248125081E-6,
59.5571980324285));
#41421=CARTESIAN_POINT('Ctrl Pts',(-1.01653186425065,-0.165518104830062,
59.5649750429453));
#41422=CARTESIAN_POINT('Ctrl Pts',(-0.933274376543597,-0.499743194453076,
59.5806771752278));
#41423=CARTESIAN_POINT('Ctrl Pts',(-0.584322219507429,-0.883741777366003,
59.604304429276));
#41424=CARTESIAN_POINT('Ctrl Pts',(-0.0912665108790651,-1.05551049774341,
59.6280797945731));
#41425=CARTESIAN_POINT('Ctrl Pts',(0.423955377218644,-0.970924212970794,
59.6518551598703));
#41426=CARTESIAN_POINT('Ctrl Pts',(0.836209932593474,-0.65052664940127,
59.6756305251674));
#41427=CARTESIAN_POINT('Ctrl Pts',(1.04537170665504,-0.172133722736198,
59.6994058904646));
#41428=CARTESIAN_POINT('Ctrl Pts',(1.00064083593713,0.348065833975191,59.7231812557618));
#41429=CARTESIAN_POINT('Ctrl Pts',(0.712881489585019,0.783729605291864,
59.7469566210589));
#41430=CARTESIAN_POINT('Ctrl Pts',(0.251982109139772,1.02904659423647,59.7707319863561));
#41431=CARTESIAN_POINT('Ctrl Pts',(-0.270116136119136,1.02443598919684,
59.7945073516532));
#41432=CARTESIAN_POINT('Ctrl Pts',(-0.726612165168123,0.7710174527789,59.8182827169504));
#41433=CARTESIAN_POINT('Ctrl Pts',(-0.97272844382277,0.383692432411846,
59.8391796105421));
#41434=CARTESIAN_POINT('Ctrl Pts',(-1.01634367445722,0.107435688288931,
59.8521513823682));
#41435=CARTESIAN_POINT('Ctrl Pts',(-1.01641695750709,-1.90763918375067E-5,
59.8571980324285));
#41436=CARTESIAN_POINT('',(-0.421648628688828,0.924896675066913,59.861775));
#41437=CARTESIAN_POINT('Origin',(0.,0.,59.861775));
#41438=CARTESIAN_POINT('Ctrl Pts',(-1.01643175349457,-2.29197629572769E-5,
59.6163519675715));
#41439=CARTESIAN_POINT('Ctrl Pts',(-1.01647698496138,-0.0544533717263767,
59.6189084273905));
#41440=CARTESIAN_POINT('Ctrl Pts',(-0.998858358818543,-0.277591283531375,
59.6293900089752));
#41441=CARTESIAN_POINT('Ctrl Pts',(-0.837879849628336,-0.648374486381346,
59.6477967123256));
#41442=CARTESIAN_POINT('Ctrl Pts',(-0.426450165346835,-0.969830983982369,
59.6715720776227));
#41443=CARTESIAN_POINT('Ctrl Pts',(0.0885519692748135,-1.0557416239719,
59.6953474429199));
#41444=CARTESIAN_POINT('Ctrl Pts',(0.582048910852398,-0.885241334592178,
59.7191228082171));
#41445=CARTESIAN_POINT('Ctrl Pts',(0.93417826195316,-0.499739406633171,
59.7428981735142));
#41446=CARTESIAN_POINT('Ctrl Pts',(1.05942882546267,0.00713467400835743,
59.7666735388114));
#41447=CARTESIAN_POINT('Ctrl Pts',(0.927356096326115,0.51227749022626,59.7904489041085));
#41448=CARTESIAN_POINT('Ctrl Pts',(0.570091202696139,0.892995264566529,
59.8142242694056));
#41449=CARTESIAN_POINT('Ctrl Pts',(0.0742928706965789,1.05682828433461,
59.8379996347028));
#41450=CARTESIAN_POINT('Ctrl Pts',(-0.268131168947707,0.994883332089929,
59.8538498782343));
#41451=CARTESIAN_POINT('Ctrl Pts',(-0.421648628688828,0.924896675066913,
59.861775));
#41452=CARTESIAN_POINT('Origin',(0.,0.,55.5071980324285));
#41453=CARTESIAN_POINT('',(-1.01640413103388,1.46689242105851E-5,59.2571980324285));
#41454=CARTESIAN_POINT('',(-1.01655516419051,1.02265252880131E-5,59.3163519675715));
#41455=CARTESIAN_POINT('',(-1.016475,-7.2179708060976E-14,55.5071980324285));
#41456=CARTESIAN_POINT('Ctrl Pts',(-1.01640413103388,1.466892421053E-5,
59.2571980324285));
#41457=CARTESIAN_POINT('Ctrl Pts',(-1.01635229931583,-0.101136172511406,
59.2619484599909));
#41458=CARTESIAN_POINT('Ctrl Pts',(-0.97631632561138,-0.371076743491578,
59.2746240093191));
#41459=CARTESIAN_POINT('Ctrl Pts',(-0.740834982929712,-0.75736088781519,
59.295224680413));
#41460=CARTESIAN_POINT('Ctrl Pts',(-0.289135652993162,-1.01923135768715,
59.3190000457102));
#41461=CARTESIAN_POINT('Ctrl Pts',(0.232786921381965,-1.0335580465354,59.3427754110073));
#41462=CARTESIAN_POINT('Ctrl Pts',(0.698171837004391,-0.796861388410206,
59.3665507763045));
#41463=CARTESIAN_POINT('Ctrl Pts',(0.993989661666965,-0.36662861157061,
59.3903261416016));
#41464=CARTESIAN_POINT('Ctrl Pts',(1.04839423183335,0.152648357301901,59.4141015068988));
#41465=CARTESIAN_POINT('Ctrl Pts',(0.848172146135856,0.634851161168593,
59.4378768721959));
#41466=CARTESIAN_POINT('Ctrl Pts',(0.441951943904046,0.962865756797002,
59.4616522374931));
#41467=CARTESIAN_POINT('Ctrl Pts',(-0.0716064543484882,1.05702625417764,
59.4854276027902));
#41468=CARTESIAN_POINT('Ctrl Pts',(-0.567773577890534,0.894463610514046,
59.5092029680874));
#41469=CARTESIAN_POINT('Ctrl Pts',(-0.926043827475508,0.514659903303883,
59.5329783333845));
#41470=CARTESIAN_POINT('Ctrl Pts',(-1.01578073897235,0.174981389455853,
59.5489766881649));
#41471=CARTESIAN_POINT('Ctrl Pts',(-1.01656332437151,0.00315563151131057,
59.5570499211796));
#41472=CARTESIAN_POINT('Ctrl Pts',(-1.01656273641868,3.31682248125081E-6,
59.5571980324285));
#41473=CARTESIAN_POINT('Ctrl Pts',(-1.01655516419051,1.02265252880044E-5,
59.3163519675715));
#41474=CARTESIAN_POINT('Ctrl Pts',(-1.01647249299314,-0.158661120223924,
59.3238069662019));
#41475=CARTESIAN_POINT('Ctrl Pts',(-0.938544820984173,-0.486088226810543,
59.339187086598));
#41476=CARTESIAN_POINT('Ctrl Pts',(-0.602081804228732,-0.871739348642251,
59.3624923287598));
#41477=CARTESIAN_POINT('Ctrl Pts',(-0.112602098016971,-1.05344803311272,
59.3862676940569));
#41478=CARTESIAN_POINT('Ctrl Pts',(0.404225617853905,-0.979302629822281,
59.4100430593541));
#41479=CARTESIAN_POINT('Ctrl Pts',(0.822877844024298,-0.667311055587846,
59.4338184246512));
#41480=CARTESIAN_POINT('Ctrl Pts',(1.04167525640482,-0.193247641021974,
59.4575937899483));
#41481=CARTESIAN_POINT('Ctrl Pts',(1.00747787145168,0.327750408428632,59.4813691552455));
#41482=CARTESIAN_POINT('Ctrl Pts',(0.728591308296158,0.769146732015046,
59.5051445205427));
#41483=CARTESIAN_POINT('Ctrl Pts',(0.272749589451039,1.02373807828526,59.5289198858398));
#41484=CARTESIAN_POINT('Ctrl Pts',(-0.24933564917612,1.02969108371093,59.552695251137));
#41485=CARTESIAN_POINT('Ctrl Pts',(-0.710863972995126,0.785559920997844,
59.5764706164341));
#41486=CARTESIAN_POINT('Ctrl Pts',(-0.968680817552861,0.397402752328119,
59.5976895219123));
#41487=CARTESIAN_POINT('Ctrl Pts',(-1.01633676570997,0.114283080288451,
59.6109833056248));
#41488=CARTESIAN_POINT('Ctrl Pts',(-1.01643175349457,-2.29197629572769E-5,
59.6163519675715));
#41489=CARTESIAN_POINT('Origin',(0.,0.,55.5071980324285));
#41490=CARTESIAN_POINT('',(-1.01648394848381,-2.59106389257236E-5,58.9571980324285));
#41491=CARTESIAN_POINT('',(-1.01639539183857,9.00667040512615E-6,59.0163519675715));
#41492=CARTESIAN_POINT('',(-1.016475,-7.2179708060976E-14,55.5071980324285));
#41493=CARTESIAN_POINT('Ctrl Pts',(-1.01648394848381,-2.59106389257809E-5,
58.9571980324285));
#41494=CARTESIAN_POINT('Ctrl Pts',(-1.01652163933797,-0.0367234553380025,
58.9589218770366));
#41495=CARTESIAN_POINT('Ctrl Pts',(-1.00561255230259,-0.242110267978689,
58.9685708434104));
#41496=CARTESIAN_POINT('Ctrl Pts',(-0.870637541598082,-0.603673966214107,
58.98614493155));
#41497=CARTESIAN_POINT('Ctrl Pts',(-0.476580245647126,-0.946204658508691,
59.0099202968471));
#41498=CARTESIAN_POINT('Ctrl Pts',(0.0332255259359154,-1.05892778353904,
59.0336956621443));
#41499=CARTESIAN_POINT('Ctrl Pts',(0.534961714244608,-0.914465937373881,
59.0574710274415));
#41500=CARTESIAN_POINT('Ctrl Pts',(0.906770144298739,-0.547905002471288,
59.0812463927386));
#41501=CARTESIAN_POINT('Ctrl Pts',(1.05834858599332,-0.0482727340283605,
59.1050217580358));
#41502=CARTESIAN_POINT('Ctrl Pts',(0.952882727939887,0.463083678311449,
59.1287971233329));
#41503=CARTESIAN_POINT('Ctrl Pts',(0.615987379842406,0.861969566863883,
59.15257248863));
#41504=CARTESIAN_POINT('Ctrl Pts',(0.129485326732331,1.05150631785341,59.1763478539272));
#41505=CARTESIAN_POINT('Ctrl Pts',(-0.388465216580355,0.985660571308298,
59.2001232192243));
#41506=CARTESIAN_POINT('Ctrl Pts',(-0.812068046017044,0.680424481454538,
59.2238985845215));
#41507=CARTESIAN_POINT('Ctrl Pts',(-0.99321101668419,0.303938289486403,
59.2429235222562));
#41508=CARTESIAN_POINT('Ctrl Pts',(-1.01643876999062,0.0676134241395438,
59.2540233382252));
#41509=CARTESIAN_POINT('Ctrl Pts',(-1.01640413103388,1.466892421053E-5,
59.2571980324285));
#41510=CARTESIAN_POINT('Ctrl Pts',(-1.01639539183857,9.00667040507064E-6,
59.0163519675715));
#41511=CARTESIAN_POINT('Ctrl Pts',(-1.01636604337103,-0.0942875579157628,
59.0207803832475));
#41512=CARTESIAN_POINT('Ctrl Pts',(-0.980065909154692,-0.357360013679804,
59.0331339206893));
#41513=CARTESIAN_POINT('Ctrl Pts',(-0.756005693342733,-0.742217880800317,
59.0534125798968));
#41514=CARTESIAN_POINT('Ctrl Pts',(-0.3096967726728,-1.01317318358827,59.0771879451939));
#41515=CARTESIAN_POINT('Ctrl Pts',(0.211829133326388,-1.03805607229115,
59.1009633104911));
#41516=CARTESIAN_POINT('Ctrl Pts',(0.681907461502236,-0.810823164995865,
59.1247386757882));
#41517=CARTESIAN_POINT('Ctrl Pts',(0.986368876446939,-0.386663200373609,
59.1485140410854));
#41518=CARTESIAN_POINT('Ctrl Pts',(1.0512679198866,0.131406817036291,59.1722894063825));
#41519=CARTESIAN_POINT('Ctrl Pts',(0.860842366221901,0.617561666122401,
59.1960647716797));
#41520=CARTESIAN_POINT('Ctrl Pts',(0.461341441599518,0.953727458558869,
59.2198401369768));
#41521=CARTESIAN_POINT('Ctrl Pts',(-0.0502068645469796,1.05825859868873,
59.243615502274));
#41522=CARTESIAN_POINT('Ctrl Pts',(-0.549561278709315,0.905767294557619,
59.2673908675711));
#41523=CARTESIAN_POINT('Ctrl Pts',(-0.91544209454521,0.533289567195347,
59.2911662328683));
#41524=CARTESIAN_POINT('Ctrl Pts',(-1.01397691023297,0.188697018515519,
59.3074865995351));
#41525=CARTESIAN_POINT('Ctrl Pts',(-1.01656037755733,0.0100162741080625,
59.3158818444361));
#41526=CARTESIAN_POINT('Ctrl Pts',(-1.01655516419051,1.02265252880044E-5,
59.3163519675715));
#41527=CARTESIAN_POINT('Origin',(0.,0.,55.5071980324285));
#41528=CARTESIAN_POINT('',(-1.01651187699763,2.32118305695883E-5,58.6571980324285));
#41529=CARTESIAN_POINT('',(-1.01650544524628,-2.41045256057504E-5,58.7163519675715));
#41530=CARTESIAN_POINT('',(-1.016475,-7.2179708060976E-14,55.5071980324285));
#41531=CARTESIAN_POINT('Ctrl Pts',(-1.01651187699763,2.32118305695597E-5,
58.6571980324285));
#41532=CARTESIAN_POINT('Ctrl Pts',(-1.01637337542594,-0.140944227048892,
58.663820415848));
#41533=CARTESIAN_POINT('Ctrl Pts',(-0.951395035985954,-0.450733549321653,
58.6783679210332));
#41534=CARTESIAN_POINT('Ctrl Pts',(-0.646842124418696,-0.839063318470144,
58.7008405479841));
#41535=CARTESIAN_POINT('Ctrl Pts',(-0.167533788876386,-1.04611873891511,
58.7246159132813));
#41536=CARTESIAN_POINT('Ctrl Pts',(0.352463981145058,-0.999100159303358,
58.7483912785784));
#41537=CARTESIAN_POINT('Ctrl Pts',(0.786857765467602,-0.709427123281846,
58.7721666438756));
#41538=CARTESIAN_POINT('Ctrl Pts',(1.03014504102483,-0.247453391119582,
58.7959420091728));
#41539=CARTESIAN_POINT('Ctrl Pts',(1.0232378965077,0.274620089350941,58.8197173744699));
#41540=CARTESIAN_POINT('Ctrl Pts',(0.767813890850171,0.729995763920686,
58.8434927397671));
#41541=CARTESIAN_POINT('Ctrl Pts',(0.325908619452451,1.00807517482141,58.8672681050642));
#41542=CARTESIAN_POINT('Ctrl Pts',(-0.195151057192915,1.04132034033774,
58.8910434703614));
#41543=CARTESIAN_POINT('Ctrl Pts',(-0.66881381045679,0.821656907271453,
58.9148188356585));
#41544=CARTESIAN_POINT('Ctrl Pts',(-0.95747415469737,0.432831070855505,
58.9368703563476));
#41545=CARTESIAN_POINT('Ctrl Pts',(-1.01634836118557,0.131988103044408,
58.9509967552709));
#41546=CARTESIAN_POINT('Ctrl Pts',(-1.01648394848381,-2.59106389257809E-5,
58.9571980324285));
#41547=CARTESIAN_POINT('Ctrl Pts',(-1.01650544524628,-2.41045256058059E-5,
58.7163519675715));
#41548=CARTESIAN_POINT('Ctrl Pts',(-1.01653538170935,-0.0298647776898298,
58.7177538002932));
#41549=CARTESIAN_POINT('Ctrl Pts',(-1.00796629632303,-0.228389592496974,
58.7270807547806));
#41550=CARTESIAN_POINT('Ctrl Pts',(-0.882672410895779,-0.585936349776809,
58.7443328310337));
#41551=CARTESIAN_POINT('Ctrl Pts',(-0.495625581575281,-0.936369197397321,
58.7681081963309));
#41552=CARTESIAN_POINT('Ctrl Pts',(0.0117953213153582,-1.05938324573377,
58.7918835616281));
#41553=CARTESIAN_POINT('Ctrl Pts',(0.516351459091809,-0.925101703403523,
58.8156589269252));
#41554=CARTESIAN_POINT('Ctrl Pts',(0.895499767177114,-0.566137931896525,
58.8394342922223));
#41555=CARTESIAN_POINT('Ctrl Pts',(1.05715535724409,-0.0696745405184991,
58.8632096575195));
#41556=CARTESIAN_POINT('Ctrl Pts',(0.962056450613156,0.443710915777326,
58.8869850228166));
#41557=CARTESIAN_POINT('Ctrl Pts',(0.633300004359957,0.84933096930703,58.9107603881138));
#41558=CARTESIAN_POINT('Ctrl Pts',(0.150732083980457,1.04867145942151,58.934535753411));
#41559=CARTESIAN_POINT('Ctrl Pts',(-0.368444590347487,0.993317962582985,
58.9583111187081));
#41560=CARTESIAN_POINT('Ctrl Pts',(-0.798136020423016,0.696714348818546,
58.9820864840053));
#41561=CARTESIAN_POINT('Ctrl Pts',(-0.990052970920145,0.31766096707036,
59.0014334336264));
#41562=CARTESIAN_POINT('Ctrl Pts',(-1.01641856558121,0.0744661931108326,
59.0128552614818));
#41563=CARTESIAN_POINT('Ctrl Pts',(-1.01639539183857,9.00667040507064E-6,
59.0163519675715));
#41564=CARTESIAN_POINT('Origin',(0.,0.,55.5071980324285));
#41565=CARTESIAN_POINT('',(-1.0163935740239,-7.14493009090905E-6,58.3571980324285));
#41566=CARTESIAN_POINT('',(-1.01649061196631,2.55351377537877E-5,58.4163519675715));
#41567=CARTESIAN_POINT('',(-1.016475,-7.2179708060976E-14,55.5071980324285));
#41568=CARTESIAN_POINT('Ctrl Pts',(-1.0163935740239,-7.14493009100481E-6,
58.3571980324285));
#41569=CARTESIAN_POINT('Ctrl Pts',(-1.01641243716347,-0.0765747908146764,
58.3607938328937));
#41570=CARTESIAN_POINT('Ctrl Pts',(-0.989051004929182,-0.321883779780578,
58.3723147551245));
#41571=CARTESIAN_POINT('Ctrl Pts',(-0.793782635482674,-0.701670231612259,
58.3917607991211));
#41572=CARTESIAN_POINT('Ctrl Pts',(-0.362252808929985,-0.995592732369494,
58.4155361644183));
#41573=CARTESIAN_POINT('Ctrl Pts',(0.157258445325715,-1.04771263603068,
58.4393115297154));
#41574=CARTESIAN_POINT('Ctrl Pts',(0.63857586865163,-0.845371425055543,
58.4630868950126));
#41575=CARTESIAN_POINT('Ctrl Pts',(0.964800452845084,-0.437712317069721,
58.4868622603097));
#41576=CARTESIAN_POINT('Ctrl Pts',(1.0567010533528,0.0762552959977839,58.5106376256069));
#41577=CARTESIAN_POINT('Ctrl Pts',(0.891957495313147,0.571702556299444,
58.534412990904));
#41578=CARTESIAN_POINT('Ctrl Pts',(0.51058154146171,0.928298699688416,58.5581883562012));
#41579=CARTESIAN_POINT('Ctrl Pts',(0.00519911514345259,1.059436149811,58.5819637214983));
#41580=CARTESIAN_POINT('Ctrl Pts',(-0.501446035884838,0.93326516029476,
58.6057390867955));
#41581=CARTESIAN_POINT('Ctrl Pts',(-0.886303482123542,0.580429258308285,
58.6295144520927));
#41582=CARTESIAN_POINT('Ctrl Pts',(-1.00866188976917,0.224167479511998,
58.6466674339703));
#41583=CARTESIAN_POINT('Ctrl Pts',(-1.01653912267294,0.0277539662379626,
58.6558952940823));
#41584=CARTESIAN_POINT('Ctrl Pts',(-1.01651187699763,2.32118305695597E-5,
58.6571980324285));
#41585=CARTESIAN_POINT('Ctrl Pts',(-1.01649061196631,2.55351377537773E-5,
58.4163519675715));
#41586=CARTESIAN_POINT('Ctrl Pts',(-1.01635293586417,-0.134095487665188,
58.4226523391046));
#41587=CARTESIAN_POINT('Ctrl Pts',(-0.956068712269705,-0.437044966876974,
58.4368778324033));
#41588=CARTESIAN_POINT('Ctrl Pts',(-0.66368501246902,-0.825805179912512,
58.4590284474679));
#41589=CARTESIAN_POINT('Ctrl Pts',(-0.188663761430564,-1.0425152162291,
58.482803812765));
#41590=CARTESIAN_POINT('Ctrl Pts',(0.33217882398349,-1.00602645086662,58.5065791780622));
#41591=CARTESIAN_POINT('Ctrl Pts',(0.772344140743365,-0.725201019859825,
58.5303545433593));
#41592=CARTESIAN_POINT('Ctrl Pts',(1.02492791636524,-0.268243839074722,
58.5541299086565));
#41593=CARTESIAN_POINT('Ctrl Pts',(1.02858437064807,0.253862528556006,58.5779052739536));
#41594=CARTESIAN_POINT('Ctrl Pts',(0.782425449558309,0.714312541419944,
58.6016806392508));
#41595=CARTESIAN_POINT('Ctrl Pts',(0.346236509580231,1.00127532196696,58.625456004548));
#41596=CARTESIAN_POINT('Ctrl Pts',(-0.174043931374068,1.04505535781517,
58.6492313698451));
#41597=CARTESIAN_POINT('Ctrl Pts',(-0.652053799988115,0.83501966016819,
58.6730067351423));
#41598=CARTESIAN_POINT('Ctrl Pts',(-0.952850717014485,0.44652188822276,
58.6953802677177));
#41599=CARTESIAN_POINT('Ctrl Pts',(-1.01636613889499,0.13883649796031,58.7098286785275));
#41600=CARTESIAN_POINT('Ctrl Pts',(-1.01650544524628,-2.41045256058059E-5,
58.7163519675715));
#41601=CARTESIAN_POINT('Origin',(0.,0.,55.5071980324285));
#41602=CARTESIAN_POINT('',(-1.0165515244855,-1.2203389089734E-5,58.0571980324285));
#41603=CARTESIAN_POINT('',(-1.01640099228082,-1.30015508006398E-5,58.1163519675715));
#41604=CARTESIAN_POINT('',(-1.016475,-7.2179708060976E-14,55.5071980324285));
#41605=CARTESIAN_POINT('Ctrl Pts',(-1.0165515244855,-1.22033890897957E-5,
58.0571980324285));
#41606=CARTESIAN_POINT('Ctrl Pts',(-1.01655885755325,-0.0121274903681481,
58.0577672499393));
#41607=CARTESIAN_POINT('Ctrl Pts',(-1.01339368204511,-0.192918087923177,
58.0662615892159));
#41608=CARTESIAN_POINT('Ctrl Pts',(-0.912103957994839,-0.538978994149835,
58.0826810502581));
#41609=CARTESIAN_POINT('Ctrl Pts',(-0.543911098024301,-0.909171438052593,
58.1064564155553));
#41610=CARTESIAN_POINT('Ctrl Pts',(-0.0436169160818455,-1.0585506841697,
58.1302317808524));
#41611=CARTESIAN_POINT('Ctrl Pts',(0.467270637269431,-0.950836546347711,
58.1540071461496));
#41612=CARTESIAN_POINT('Ctrl Pts',(0.864670767536001,-0.612189880750512,
58.1777825114467));
#41613=CARTESIAN_POINT('Ctrl Pts',(1.05206571151958,-0.124858820150662,
58.2015578767439));
#41614=CARTESIAN_POINT('Ctrl Pts',(0.983942296348724,0.392797077102948,
58.2253332420411));
#41615=CARTESIAN_POINT('Ctrl Pts',(0.676845860469362,0.815053168505043,
58.2491086073382));
#41616=CARTESIAN_POINT('Ctrl Pts',(0.205361837603814,1.03935484892341,58.2728839726354));
#41617=CARTESIAN_POINT('Ctrl Pts',(-0.315999031548909,1.01122529556216,
58.2966593379325));
#41618=CARTESIAN_POINT('Ctrl Pts',(-0.760612266830792,0.737496417531059,
58.3204347032296));
#41619=CARTESIAN_POINT('Ctrl Pts',(-0.981188751078297,0.353138397649337,
58.3406142680616));
#41620=CARTESIAN_POINT('Ctrl Pts',(-1.01637086292167,0.09217982247098,58.3528687111279));
#41621=CARTESIAN_POINT('Ctrl Pts',(-1.0163935740239,-7.14493009100481E-6,
58.3571980324285));
#41622=CARTESIAN_POINT('Ctrl Pts',(-1.01640099228083,-1.3001550800619E-5,
58.1163519675715));
#41623=CARTESIAN_POINT('Ctrl Pts',(-1.01643252806871,-0.0697223898558531,
58.1196257561502));
#41624=CARTESIAN_POINT('Ctrl Pts',(-0.992255076331624,-0.308161297059955,
58.1308246664947));
#41625=CARTESIAN_POINT('Ctrl Pts',(-0.807815818999105,-0.685467427031471,
58.1499486986049));
#41626=CARTESIAN_POINT('Ctrl Pts',(-0.382320725410081,-0.988060146887956,
58.173724063902));
#41627=CARTESIAN_POINT('Ctrl Pts',(0.136029751029905,-1.05067973130782,
58.1974994291992));
#41628=CARTESIAN_POINT('Ctrl Pts',(0.62134227328246,-0.858117573749964,
58.2212747944964));
#41629=CARTESIAN_POINT('Ctrl Pts',(0.955747531469626,-0.457141823765944,
58.2450501597935));
#41630=CARTESIAN_POINT('Ctrl Pts',(1.05802751617526,0.0548613339460823,
58.2688255250907));
#41631=CARTESIAN_POINT('Ctrl Pts',(0.903341180323916,0.553540154710871,
58.2926008903878));
#41632=CARTESIAN_POINT('Ctrl Pts',(0.5292576588922,0.917779015586153,58.316376255685));
#41633=CARTESIAN_POINT('Ctrl Pts',(0.0266317402610465,1.05911413046801,
58.3401516209821));
#41634=CARTESIAN_POINT('Ctrl Pts',(-0.482462309113668,0.94321901551604,
58.3639269862793));
#41635=CARTESIAN_POINT('Ctrl Pts',(-0.874379288435858,0.598241465380611,
58.3877023515764));
#41636=CARTESIAN_POINT('Ctrl Pts',(-1.00635212941563,0.237887822759668,
58.4051773453405));
#41637=CARTESIAN_POINT('Ctrl Pts',(-1.01652611610726,0.0346128863531156,
58.4147272173389));
#41638=CARTESIAN_POINT('Ctrl Pts',(-1.01649061196631,2.55351377537773E-5,
58.4163519675715));
#41639=CARTESIAN_POINT('Origin',(0.,0.,55.5071980324285));
#41640=CARTESIAN_POINT('',(-1.01643729572907,2.38158822067048E-5,57.7571980324285));
#41641=CARTESIAN_POINT('',(-1.01656116828543,-5.50351341488398E-6,57.8163519675715));
#41642=CARTESIAN_POINT('',(-1.016475,-7.2179708060976E-14,55.5071980324285));
#41643=CARTESIAN_POINT('Ctrl Pts',(-1.01643729572907,2.38158822067069E-5,
57.7571980324285));
#41644=CARTESIAN_POINT('Ctrl Pts',(-1.01633594492437,-0.116390217672064,
57.7626657887507));
#41645=CARTESIAN_POINT('Ctrl Pts',(-0.967402991324987,-0.401621088357726,
57.7760586668386));
#41646=CARTESIAN_POINT('Ctrl Pts',(-0.705959114011145,-0.789970705576619,
57.7973766666922));
#41647=CARTESIAN_POINT('Ctrl Pts',(-0.242919704987064,-1.03122354669277,
57.8211520319894));
#41648=CARTESIAN_POINT('Ctrl Pts',(0.2791183423777,-1.02202002782379,57.8449273972865));
#41649=CARTESIAN_POINT('Ctrl Pts',(0.73336607961892,-0.764595435239446,
57.8687027625837));
#41650=CARTESIAN_POINT('Ctrl Pts',(1.00949899449501,-0.321471252895473,
57.8924781278809));
#41651=CARTESIAN_POINT('Ctrl Pts',(1.04045185662625,0.199729618153172,57.916253493178));
#41652=CARTESIAN_POINT('Ctrl Pts',(0.818707051422304,0.672421556968558,
57.9400288584752));
#41653=CARTESIAN_POINT('Ctrl Pts',(0.398120405716357,0.981800452677053,
57.9638042237723));
#41654=CARTESIAN_POINT('Ctrl Pts',(-0.11915893864965,1.05272652368244,57.9875795890695));
#41655=CARTESIAN_POINT('Ctrl Pts',(-0.607497793701196,0.867973742098689,
58.0113549543666));
#41656=CARTESIAN_POINT('Ctrl Pts',(-0.940132720180615,0.481883868106556,
58.034561102153));
#41657=CARTESIAN_POINT('Ctrl Pts',(-1.01645676045732,0.156551657251636,
58.0498421281736));
#41658=CARTESIAN_POINT('Ctrl Pts',(-1.0165515244855,-1.22033890897957E-5,
58.0571980324285));
#41659=CARTESIAN_POINT('Ctrl Pts',(-1.01656116828543,-5.50351341484581E-6,
57.8163519675715));
#41660=CARTESIAN_POINT('Ctrl Pts',(-1.01656274467139,-0.00526690962334575,
57.8165991731959));
#41661=CARTESIAN_POINT('Ctrl Pts',(-1.01524049810908,-0.179202016646892,
57.824771500586));
#41662=CARTESIAN_POINT('Ctrl Pts',(-0.922821481937435,-0.520415702512074,
57.8408689497419));
#41663=CARTESIAN_POINT('Ctrl Pts',(-0.562193425992196,-0.897981371030322,
57.864644315039));
#41664=CARTESIAN_POINT('Ctrl Pts',(-0.0650237641719233,-1.05745160694911,
57.8884196803362));
#41665=CARTESIAN_POINT('Ctrl Pts',(0.447938414546611,-0.960095395114365,
57.9121950456334));
#41666=CARTESIAN_POINT('Ctrl Pts',(0.852108445175959,-0.629557931096218,
57.9359704109305));
#41667=CARTESIAN_POINT('Ctrl Pts',(1.04932433848386,-0.146117841524369,
57.9597457762276));
#41668=CARTESIAN_POINT('Ctrl Pts',(0.991687678140017,0.372810327072094,
57.9835211415248));
#41669=CARTESIAN_POINT('Ctrl Pts',(0.693196852949359,0.80119293182569,58.007296506822));
#41670=CARTESIAN_POINT('Ctrl Pts',(0.226347226119961,1.03498740290602,58.0310718721191));
#41671=CARTESIAN_POINT('Ctrl Pts',(-0.295476031333513,1.01741137493825,
58.0548472374163));
#41672=CARTESIAN_POINT('Ctrl Pts',(-0.745536137617694,0.752733590623157,
58.0786226027134));
#41673=CARTESIAN_POINT('Ctrl Pts',(-0.977486684416592,0.366855908733197,
58.0991241794318));
#41674=CARTESIAN_POINT('Ctrl Pts',(-1.01635618686555,0.0990286999729323,
58.1117006343845));
#41675=CARTESIAN_POINT('Ctrl Pts',(-1.01640099228083,-1.3001550800619E-5,
58.1163519675715));
#41676=CARTESIAN_POINT('Origin',(0.,0.,55.5071980324285));
#41677=CARTESIAN_POINT('',(-1.01643822360686,-2.39497420581337E-5,57.4571980324285));
#41678=CARTESIAN_POINT('',(-1.0164203332823,2.04341709851841E-5,57.5163519675715));
#41679=CARTESIAN_POINT('',(-1.016475,-7.2179708060976E-14,55.5071980324285));
#41680=CARTESIAN_POINT('Ctrl Pts',(-1.01643822360686,-2.39497420582019E-5,
57.4571980324285));
#41681=CARTESIAN_POINT('Ctrl Pts',(-1.01648379076976,-0.0519988508214108,
57.4596392057963));
#41682=CARTESIAN_POINT('Ctrl Pts',(-0.999851515608375,-0.272678234287765,
57.4700055009299));
#41683=CARTESIAN_POINT('Ctrl Pts',(-0.842554347220154,-0.642288220587176,
57.4882969178293));
#41684=CARTESIAN_POINT('Ctrl Pts',(-0.433464221124387,-0.966716481358237,
57.5120722831264));
#41685=CARTESIAN_POINT('Ctrl Pts',(0.0809026622319955,-1.05635540684393,
57.5358476484236));
#41686=CARTESIAN_POINT('Ctrl Pts',(0.575620473027226,-0.889434121987983,
57.5596230137207));
#41687=CARTESIAN_POINT('Ctrl Pts',(0.930535610706933,-0.506493300578492,
57.5833983790179));
#41688=CARTESIAN_POINT('Ctrl Pts',(1.05944876982279,-0.000538930044200919,
57.607173744315));
#41689=CARTESIAN_POINT('Ctrl Pts',(0.931050424239669,0.505546332048563,
57.6309491096122));
#41690=CARTESIAN_POINT('Ctrl Pts',(0.576525065783793,0.888848038107536,
57.6547244749094));
#41691=CARTESIAN_POINT('Ctrl Pts',(0.0819773330527327,1.05627255156526,
57.6784998402065));
#41692=CARTESIAN_POINT('Ctrl Pts',(-0.432480480769399,0.967156977991728,
57.7022752055036));
#41693=CARTESIAN_POINT('Ctrl Pts',(-0.841900461305519,0.643145084392453,
57.7260505708008));
#41694=CARTESIAN_POINT('Ctrl Pts',(-0.999713158006665,0.273368272745295,
57.7443581797758));
#41695=CARTESIAN_POINT('Ctrl Pts',(-1.01648284566773,0.0523435986850332,
57.754740666985));
#41696=CARTESIAN_POINT('Ctrl Pts',(-1.01643729572907,2.38158822067069E-5,
57.7571980324285));
#41697=CARTESIAN_POINT('Ctrl Pts',(-1.0164203332823,2.04341709851633E-5,
57.5163519675715));
#41698=CARTESIAN_POINT('Ctrl Pts',(-1.01634044576945,-0.109542886279426,
57.5214977120073));
#41699=CARTESIAN_POINT('Ctrl Pts',(-0.971500612426874,-0.387911922967112,
57.5345685782088));
#41700=CARTESIAN_POINT('Ctrl Pts',(-0.721796698973036,-0.775526605796326,
57.555564566176));
#41701=CARTESIAN_POINT('Ctrl Pts',(-0.263732900340999,-1.02609792331145,
57.5793399314732));
#41702=CARTESIAN_POINT('Ctrl Pts',(0.258384499898145,-1.02745775638647,
57.6031152967703));
#41703=CARTESIAN_POINT('Ctrl Pts',(0.717747280609244,-0.779275838278319,
57.6268906620675));
#41704=CARTESIAN_POINT('Ctrl Pts',(1.00278862358054,-0.341828856833032,
57.6506660273646));
#41705=CARTESIAN_POINT('Ctrl Pts',(1.04427968174507,0.178639125727723,57.6744413926618));
#41706=CARTESIAN_POINT('Ctrl Pts',(0.832143397191218,0.655720487294243,
57.6982167579589));
#41707=CARTESIAN_POINT('Ctrl Pts',(0.417901946483455,0.973545044706037,
57.7219921232561));
#41708=CARTESIAN_POINT('Ctrl Pts',(-0.0978366051027944,1.05492179314312,
57.7457674885532));
#41709=CARTESIAN_POINT('Ctrl Pts',(-0.589813286563081,0.880086517303837,
57.7695428538504));
#41710=CARTESIAN_POINT('Ctrl Pts',(-0.934914336585201,0.495542314056757,
57.7930710135232));
#41711=CARTESIAN_POINT('Ctrl Pts',(-1.01651220759037,0.163407586277906,
57.8086740514302));
#41712=CARTESIAN_POINT('Ctrl Pts',(-1.01656116828543,-5.50351341484581E-6,
57.8163519675715));
#41713=CARTESIAN_POINT('Origin',(0.,0.,55.5071980324285));
#41714=CARTESIAN_POINT('',(-1.01655087939569,1.25177289053898E-5,57.1571980324285));
#41715=CARTESIAN_POINT('',(-1.01645785338958,-2.58202779849781E-5,57.2163519675715));
#41716=CARTESIAN_POINT('',(-1.016475,-7.2179708060976E-14,55.5071980324285));
#41717=CARTESIAN_POINT('Ctrl Pts',(-1.01655087939569,1.25177289053684E-5,
57.1571980324285));
#41718=CARTESIAN_POINT('Ctrl Pts',(-1.01645429891022,-0.156206996899727,
57.1645377446077));
#41719=CARTESIAN_POINT('Ctrl Pts',(-0.940390670028725,-0.481196778392105,
57.1798025785527));
#41720=CARTESIAN_POINT('Ctrl Pts',(-0.608380536643186,-0.867355238041698,
57.2029925342634));
#41721=CARTESIAN_POINT('Ctrl Pts',(-0.120229897725971,-1.05260474919004,
57.2267678995606));
#41722=CARTESIAN_POINT('Ctrl Pts',(0.397121337553111,-0.982204983485956,
57.2505432648577));
#41723=CARTESIAN_POINT('Ctrl Pts',(0.818022520857566,-0.673254143466235,
57.2743186301549));
#41724=CARTESIAN_POINT('Ctrl Pts',(1.04024811765422,-0.200788047556321,
57.298093995452));
#41725=CARTESIAN_POINT('Ctrl Pts',(1.00982552981173,0.320444044514911,57.3218693607492));
#41726=CARTESIAN_POINT('Ctrl Pts',(0.734143582611297,0.763848929065998,
57.3456447260463));
#41727=CARTESIAN_POINT('Ctrl Pts',(0.280157978558803,1.02173553005387,57.3694200913435));
#41728=CARTESIAN_POINT('Ctrl Pts',(-0.241870435179003,1.03147015415423,
57.3931954566406));
#41729=CARTESIAN_POINT('Ctrl Pts',(-0.705155049885808,0.79068852397462,
57.4169708219378));
#41730=CARTESIAN_POINT('Ctrl Pts',(-0.967192769783646,0.402310326406248,
57.4383050138671));
#41731=CARTESIAN_POINT('Ctrl Pts',(-1.01633585973001,0.116734523561822,
57.4517140840306));
#41732=CARTESIAN_POINT('Ctrl Pts',(-1.01643822360686,-2.39497420582019E-5,
57.4571980324285));
#41733=CARTESIAN_POINT('Ctrl Pts',(-1.01645785338958,-2.58202779849365E-5,
57.2163519675715));
#41734=CARTESIAN_POINT('Ctrl Pts',(-1.01650184768103,-0.0451422806476026,
57.218471129053));
#41735=CARTESIAN_POINT('Ctrl Pts',(-1.00252655417846,-0.2589557093226,57.2285154123001));
#41736=CARTESIAN_POINT('Ctrl Pts',(-0.855376177906754,-0.62511085834112,
57.246484817313));
#41737=CARTESIAN_POINT('Ctrl Pts',(-0.452933360879266,-0.957749112006351,
57.2702601826102));
#41738=CARTESIAN_POINT('Ctrl Pts',(0.0595147418551541,-1.0577759623135,
57.2940355479073));
#41739=CARTESIAN_POINT('Ctrl Pts',(0.557508320487304,-0.900897587705596,
57.3178109132045));
#41740=CARTESIAN_POINT('Ctrl Pts',(0.920098178889751,-0.525215510195677,
57.3415862785016));
#41741=CARTESIAN_POINT('Ctrl Pts',(1.0592210291418,-0.0219727642805258,
57.3653616437988));
#41742=CARTESIAN_POINT('Ctrl Pts',(0.941087686758059,0.486606572888925,
57.3891370090959));
#41743=CARTESIAN_POINT('Ctrl Pts',(0.594389551407591,0.877002310215783,
57.4129123743931));
#41744=CARTESIAN_POINT('Ctrl Pts',(0.103330240503893,1.05439786245219,57.4366877396903));
#41745=CARTESIAN_POINT('Ctrl Pts',(-0.412825196255343,0.975708639032718,
57.4604631049874));
#41746=CARTESIAN_POINT('Ctrl Pts',(-0.828716537711619,0.660046127986225,
57.4842384702846));
#41747=CARTESIAN_POINT('Ctrl Pts',(-0.996884749609738,0.287091239458341,
57.5028680911459));
#41748=CARTESIAN_POINT('Ctrl Pts',(-1.01646348302378,0.0591990064556959,
57.5135725902416));
#41749=CARTESIAN_POINT('Ctrl Pts',(-1.0164203332823,2.04341709851633E-5,
57.5163519675715));
#41750=CARTESIAN_POINT('Origin',(0.,0.,55.5071980324285));
#41751=CARTESIAN_POINT('',(-1.01639331761686,6.83678408873587E-6,56.8571980324285));
#41752=CARTESIAN_POINT('',(-1.01653552617529,1.81671041117951E-5,56.9163519675715));
#41753=CARTESIAN_POINT('',(-1.016475,-7.2179708060976E-14,55.5071980324285));
#41754=CARTESIAN_POINT('Ctrl Pts',(-1.01639331761686,6.83678408874844E-6,
56.8571980324285));
#41755=CARTESIAN_POINT('Ctrl Pts',(-1.01637167394885,-0.0918354088346601,
56.8615111616534));
#41756=CARTESIAN_POINT('Ctrl Pts',(-0.981370841868257,-0.352448563742444,
56.873749412644));
#41757=CARTESIAN_POINT('Ctrl Pts',(-0.761362185779602,-0.736722205712254,
56.8939127854004));
#41758=CARTESIAN_POINT('Ctrl Pts',(-0.317027666320693,-1.01090328177916,
56.9176881506975));
#41759=CARTESIAN_POINT('Ctrl Pts',(0.204304314625503,-1.03956324163084,
56.9414635159947));
#41760=CARTESIAN_POINT('Ctrl Pts',(0.676016293066456,-0.815741354740158,
56.9652388812919));
#41761=CARTESIAN_POINT('Ctrl Pts',(0.98354216404791,-0.393797915007909,
56.989014246589));
#41762=CARTESIAN_POINT('Ctrl Pts',(1.05219219565452,0.123788407083776,57.0127896118862));
#41763=CARTESIAN_POINT('Ctrl Pts',(0.865293148524952,0.611309866958155,
57.0365649771833));
#41764=CARTESIAN_POINT('Ctrl Pts',(0.468237755572337,0.950360663422683,
57.0603403424805));
#41765=CARTESIAN_POINT('Ctrl Pts',(-0.0425399473918753,1.05859451122728,
57.0841157077776));
#41766=CARTESIAN_POINT('Ctrl Pts',(-0.54298584556759,0.90972433068368,57.1078910730748));
#41767=CARTESIAN_POINT('Ctrl Pts',(-0.911555140614478,0.539906669660545,
57.1316664383719));
#41768=CARTESIAN_POINT('Ctrl Pts',(-1.01329712113469,0.193607825789528,
57.1481020914898));
#41769=CARTESIAN_POINT('Ctrl Pts',(-1.01655858257814,0.0124724615555045,
57.156612622842));
#41770=CARTESIAN_POINT('Ctrl Pts',(-1.01655087939569,1.25177289053684E-5,
57.1571980324285));
#41771=CARTESIAN_POINT('Ctrl Pts',(-1.01653552617529,1.81671041117881E-5,
56.9163519675715));
#41772=CARTESIAN_POINT('Ctrl Pts',(-1.01641141768326,-0.14935414160094,
56.9233696678643));
#41773=CARTESIAN_POINT('Ctrl Pts',(-0.94543258794415,-0.46752734399196,
56.9383124899229));
#41774=CARTESIAN_POINT('Ctrl Pts',(-0.62580367676965,-0.854869433941773,
56.9611804337472));
#41775=CARTESIAN_POINT('Ctrl Pts',(-0.141500771893025,-1.04995691459222,
56.9849557990443));
#41776=CARTESIAN_POINT('Ctrl Pts',(0.377168850439841,-0.990038205931583,
57.0087311643415));
#41777=CARTESIAN_POINT('Ctrl Pts',(0.804234341269022,-0.689665944693458,
57.0325065296386));
#41778=CARTESIAN_POINT('Ctrl Pts',(1.0359730221788,-0.221792444109516,57.0562818949358));
#41779=CARTESIAN_POINT('Ctrl Pts',(1.01610182372747,0.29994845351169,57.0800572602329));
#41780=CARTESIAN_POINT('Ctrl Pts',(0.749446923564514,0.748839969356621,
57.1038326255301));
#41781=CARTESIAN_POINT('Ctrl Pts',(0.300771598169799,1.0158584727612,57.1276079908272));
#41782=CARTESIAN_POINT('Ctrl Pts',(-0.220953028616557,1.03615237783422,
57.1513833561244));
#41783=CARTESIAN_POINT('Ctrl Pts',(-0.689014129727543,0.804792842899423,
57.1751587214215));
#41784=CARTESIAN_POINT('Ctrl Pts',(-0.962928490231453,0.416014631120328,
57.1968149252373));
#41785=CARTESIAN_POINT('Ctrl Pts',(-1.01633732028666,0.123581738355737,
57.2105460072872));
#41786=CARTESIAN_POINT('Ctrl Pts',(-1.01645785338958,-2.58202779849365E-5,
57.2163519675715));
#41787=CARTESIAN_POINT('Origin',(0.,0.,55.5071980324285));
#41788=CARTESIAN_POINT('',(-1.0165129144013,-2.30512370967894E-5,56.5571980324285));
#41789=CARTESIAN_POINT('',(-1.01639061276947,5.63170237111166E-7,56.6163519675715));
#41790=CARTESIAN_POINT('',(-1.016475,-7.2179708060976E-14,55.5071980324285));
#41791=CARTESIAN_POINT('Ctrl Pts',(-1.0165129144013,-2.30512370968383E-5,
56.5571980324285));
#41792=CARTESIAN_POINT('Ctrl Pts',(-1.01653971143184,-0.0274090521408874,
56.5584845786991));
#41793=CARTESIAN_POINT('Ctrl Pts',(-1.00877426909957,-0.223477594555612,
56.5676962467354));
#41794=CARTESIAN_POINT('Ctrl Pts',(-0.886893539358715,-0.579527252302758,
56.5848330365374));
#41795=CARTESIAN_POINT('Ctrl Pts',(-0.502395259761104,-0.932754517168359,
56.6086084018346));
#41796=CARTESIAN_POINT('Ctrl Pts',(0.00412126548291853,-1.05944089098629,
56.6323837671317));
#41797=CARTESIAN_POINT('Ctrl Pts',(0.509636846599777,-0.928817673665269,
56.6561591324289));
#41798=CARTESIAN_POINT('Ctrl Pts',(0.89137539612891,-0.572609718307843,
56.679934497726));
#41799=CARTESIAN_POINT('Ctrl Pts',(1.05662292602311,-0.0773303208768799,
56.7037098630232));
#41800=CARTESIAN_POINT('Ctrl Pts',(0.965245272389302,0.436730523841399,
56.7274852283203));
#41801=CARTESIAN_POINT('Ctrl Pts',(0.639435600411005,0.844721314547941,
56.7512605936175));
#41802=CARTESIAN_POINT('Ctrl Pts',(0.158324283665738,1.04755210253542,56.7750359589146));
#41803=CARTESIAN_POINT('Ctrl Pts',(-0.361239727368135,0.995960765138673,
56.7988113242118));
#41804=CARTESIAN_POINT('Ctrl Pts',(-0.793068360860628,0.702477445421887,
56.8225866895089));
#41805=CARTESIAN_POINT('Ctrl Pts',(-0.988885930748487,0.322573781877596,
56.8420489255812));
#41806=CARTESIAN_POINT('Ctrl Pts',(-1.01641144291832,0.0769193262567779,
56.8535860398877));
#41807=CARTESIAN_POINT('Ctrl Pts',(-1.01639331761686,6.83678408874844E-6,
56.8571980324285));
#41808=CARTESIAN_POINT('Ctrl Pts',(-1.01639061276947,5.63170237152799E-7,
56.6163519675715));
#41809=CARTESIAN_POINT('Ctrl Pts',(-1.01638896833711,-0.0849855231432444,
56.62034308491));
#41810=CARTESIAN_POINT('Ctrl Pts',(-0.984911757328215,-0.338728827146233,
56.6322593240142));
#41811=CARTESIAN_POINT('Ctrl Pts',(-0.776111149103991,-0.721168132395479,
56.6521006848841));
#41812=CARTESIAN_POINT('Ctrl Pts',(-0.337414590176968,-1.00428252264095,
56.6758760501813));
#41813=CARTESIAN_POINT('Ctrl Pts',(0.18323086366488,-1.043483800328,56.6996514154785));
#41814=CARTESIAN_POINT('Ctrl Pts',(0.659374487328757,-0.82925103340682,
56.7234267807756));
#41815=CARTESIAN_POINT('Ctrl Pts',(0.975373848875025,-0.41361557741103,
56.7472021460728));
#41816=CARTESIAN_POINT('Ctrl Pts',(1.05448123428539,0.102475936132846,56.77097751137));
#41817=CARTESIAN_POINT('Ctrl Pts',(0.877483595272346,0.593678811289621,
56.7947528766671));
#41818=CARTESIAN_POINT('Ctrl Pts',(0.48736888002166,0.940693130480272,56.8185282419642));
#41819=CARTESIAN_POINT('Ctrl Pts',(-0.02111457889448,1.0592384837724,56.8423036072614));
#41820=CARTESIAN_POINT('Ctrl Pts',(-0.524469876618518,0.920523405170176,
56.8660789725585));
#41821=CARTESIAN_POINT('Ctrl Pts',(-0.900445600203663,0.558238042433696,
56.8898543378557));
#41822=CARTESIAN_POINT('Ctrl Pts',(-1.01130302005036,0.207325373739056,
56.90661200286));
#41823=CARTESIAN_POINT('Ctrl Pts',(-1.01655157398383,0.0193327053028336,
56.9154445460986));
#41824=CARTESIAN_POINT('Ctrl Pts',(-1.01653552617529,1.81671041117881E-5,
56.9163519675715));
#41825=CARTESIAN_POINT('Origin',(0.,0.,55.5071980324285));
#41826=CARTESIAN_POINT('',(-1.01648283811887,2.60095369413545E-5,56.2571980324285));
#41827=CARTESIAN_POINT('',(-1.01653237544382,-1.90345246380841E-5,56.3163519675715));
#41828=CARTESIAN_POINT('',(-1.016475,-7.2179708060976E-14,55.5071980324285));
#41829=CARTESIAN_POINT('Ctrl Pts',(-1.01648283811887,2.60095369413633E-5,
56.2571980324285));
#41830=CARTESIAN_POINT('Ctrl Pts',(-1.01634766438916,-0.131643710346183,
56.2633831175105));
#41831=CARTESIAN_POINT('Ctrl Pts',(-0.957702373223059,-0.432142526414999,
56.2774933243581));
#41832=CARTESIAN_POINT('Ctrl Pts',(-0.669649384741906,-0.820976009905639,
56.2995286529715));
#41833=CARTESIAN_POINT('Ctrl Pts',(-0.196210379601176,-1.04112127560369,
56.3233040182687));
#41834=CARTESIAN_POINT('Ctrl Pts',(0.324882860612091,-1.00840621766713,
56.3470793835659));
#41835=CARTESIAN_POINT('Ctrl Pts',(0.767070810376454,-0.730776546609132,
56.370854748863));
#41836=CARTESIAN_POINT('Ctrl Pts',(1.02295797523586,-0.275660965237961,
56.3946301141602));
#41837=CARTESIAN_POINT('Ctrl Pts',(1.03039626118959,0.246405215445278,56.4184054794573));
#41838=CARTESIAN_POINT('Ctrl Pts',(0.787579113904559,0.708626224754583,
56.4421808447545));
#41839=CARTESIAN_POINT('Ctrl Pts',(0.353480261128564,0.998741052994776,
56.4659562100516));
#41840=CARTESIAN_POINT('Ctrl Pts',(-0.166469404010035,1.04628864277636,
56.4897315753488));
#41841=CARTESIAN_POINT('Ctrl Pts',(-0.645988145161798,0.839720967104466,
56.5135069406459));
#41842=CARTESIAN_POINT('Ctrl Pts',(-0.951155699582826,0.451421666720772,
56.5359957596725));
#41843=CARTESIAN_POINT('Ctrl Pts',(-1.01637464179167,0.141288644010153,
56.5505594569333));
#41844=CARTESIAN_POINT('Ctrl Pts',(-1.0165129144013,-2.30512370968383E-5,
56.5571980324285));
#41845=CARTESIAN_POINT('Ctrl Pts',(-1.01653237544382,-1.90345246380841E-5,
56.3163519675715));
#41846=CARTESIAN_POINT('Ctrl Pts',(-1.01655003026065,-0.0205494097757443,
56.3173165019557));
#41847=CARTESIAN_POINT('Ctrl Pts',(-1.01093463056855,-0.209758496430707,
56.3262061581056));
#41848=CARTESIAN_POINT('Ctrl Pts',(-0.898436564193858,-0.561465699584117,
56.3430209360212));
#41849=CARTESIAN_POINT('Ctrl Pts',(-0.521163199217816,-0.922399539433787,
56.3667963013183));
#41850=CARTESIAN_POINT('Ctrl Pts',(-0.0173133632032956,-1.05930743344434,
56.3905716666155));
#41851=CARTESIAN_POINT('Ctrl Pts',(0.49074142153069,-0.938938149241069,
56.4143470319126));
#41852=CARTESIAN_POINT('Ctrl Pts',(0.879608363221454,-0.590526136845567,
56.4381223972097));
#41853=CARTESIAN_POINT('Ctrl Pts',(1.05484217994403,-0.0986912679291979,
56.4618977625069));
#41854=CARTESIAN_POINT('Ctrl Pts',(0.973883308267136,0.417113045610174,
56.4856731278041));
#41855=CARTESIAN_POINT('Ctrl Pts',(0.656394472537722,0.831611861009717,
56.5094484931012));
#41856=CARTESIAN_POINT('Ctrl Pts',(0.179485139828959,1.0441346060376,56.5332238583984));
#41857=CARTESIAN_POINT('Ctrl Pts',(-0.341016287857761,1.00306524332296,
56.5569992236956));
#41858=CARTESIAN_POINT('Ctrl Pts',(-0.778694065497443,0.718378412332483,
56.5807745889927));
#41859=CARTESIAN_POINT('Ctrl Pts',(-0.985523871362989,0.336295280666352,
56.6005588369514));
#41860=CARTESIAN_POINT('Ctrl Pts',(-1.01639223367,0.0837704981166061,56.6124179631443));
#41861=CARTESIAN_POINT('Ctrl Pts',(-1.01639061276947,5.63170237152799E-7,
56.6163519675715));
#41862=CARTESIAN_POINT('Origin',(1.39932914042665E-16,0.,59.861775));
#41863=CARTESIAN_POINT('',(0.672748867539255,-0.97943229058963,59.861775));
#41864=CARTESIAN_POINT('Ctrl Pts',(-1.01184089351566,-0.0973166075163435,
59.861775));
#41865=CARTESIAN_POINT('Ctrl Pts',(-1.0114437912448,-0.126338627735325,
59.861775));
#41866=CARTESIAN_POINT('Ctrl Pts',(-1.0097970940642,-0.15529997051701,59.861775));
#41867=CARTESIAN_POINT('Ctrl Pts',(-1.00689935402508,-0.184119087090023,
59.861775));
#41868=CARTESIAN_POINT('Ctrl Pts',(-1.00255508251114,-0.227324504241121,
59.861775));
#41869=CARTESIAN_POINT('Ctrl Pts',(-0.99540135320563,-0.270210478356502,
59.861775));
#41870=CARTESIAN_POINT('Ctrl Pts',(-0.98556589048639,-0.312540257335641,
59.861775));
#41871=CARTESIAN_POINT('Ctrl Pts',(-0.981595087308391,-0.329629765546126,
59.861775));
#41872=CARTESIAN_POINT('Ctrl Pts',(-0.977186645817288,-0.346628644562582,
59.861775));
#41873=CARTESIAN_POINT('Ctrl Pts',(-0.97234684431464,-0.363521208153442,
59.861775));
#41874=CARTESIAN_POINT('Ctrl Pts',(-0.969416300323676,-0.3737498096149,
59.861775));
#41875=CARTESIAN_POINT('Ctrl Pts',(-0.966329907396498,-0.383931170219947,
59.861775));
#41876=CARTESIAN_POINT('Ctrl Pts',(-0.963090796052553,-0.394058609457477,
59.861775));
#41877=CARTESIAN_POINT('Ctrl Pts',(-0.949182573622318,-0.43754420245124,
59.861775));
#41878=CARTESIAN_POINT('Ctrl Pts',(-0.93245720400045,-0.480055494132926,
59.861775));
#41879=CARTESIAN_POINT('Ctrl Pts',(-0.91305514527965,-0.5213247168299,59.861775));
#41880=CARTESIAN_POINT('Ctrl Pts',(-0.900416920921426,-0.548206899954864,
59.861775));
#41881=CARTESIAN_POINT('Ctrl Pts',(-0.886641870555354,-0.574562125052264,
59.861775));
#41882=CARTESIAN_POINT('Ctrl Pts',(-0.87175731975576,-0.600313985396109,
59.861775));
#41883=CARTESIAN_POINT('Ctrl Pts',(-0.864826659378796,-0.612304767013991,
59.861775));
#41884=CARTESIAN_POINT('Ctrl Pts',(-0.857652040875426,-0.624169497956551,
59.861775));
#41885=CARTESIAN_POINT('Ctrl Pts',(-0.85025378976052,-0.635872550479802,
59.861775));
#41886=CARTESIAN_POINT('Ctrl Pts',(-0.843281093125467,-0.646902432229058,
59.861775));
#41887=CARTESIAN_POINT('Ctrl Pts',(-0.836107645721068,-0.657792743080534,
59.861775));
#41888=CARTESIAN_POINT('Ctrl Pts',(-0.828736935305739,-0.668537604860453,
59.861775));
#41889=CARTESIAN_POINT('Ctrl Pts',(-0.802624452178946,-0.7066038164083,
59.861775));
#41890=CARTESIAN_POINT('Ctrl Pts',(-0.774040170525397,-0.742845924874012,
59.861775));
#41891=CARTESIAN_POINT('Ctrl Pts',(-0.743254711167329,-0.777114570540984,
59.861775));
#41892=CARTESIAN_POINT('Ctrl Pts',(-0.7121921018527,-0.811691723985851,
59.861775));
#41893=CARTESIAN_POINT('Ctrl Pts',(-0.678887800198998,-0.844260574715302,
59.861775));
#41894=CARTESIAN_POINT('Ctrl Pts',(-0.643572524360008,-0.874642276826878,
59.861775));
#41895=CARTESIAN_POINT('Ctrl Pts',(-0.623233617211618,-0.892139821545903,
59.861775));
#41896=CARTESIAN_POINT('Ctrl Pts',(-0.602226877710127,-0.908911380096442,
59.861775));
#41897=CARTESIAN_POINT('Ctrl Pts',(-0.580590775824314,-0.924917292668666,
59.861775));
#41898=CARTESIAN_POINT('Ctrl Pts',(-0.573562898026258,-0.930116362177473,
59.861775));
#41899=CARTESIAN_POINT('Ctrl Pts',(-0.566476752841383,-0.935228569208567,
59.861775));
#41900=CARTESIAN_POINT('Ctrl Pts',(-0.559334318108606,-0.940252829215512,
59.861775));
#41901=CARTESIAN_POINT('Ctrl Pts',(-0.520393486038798,-0.967645290263513,
59.861775));
#41902=CARTESIAN_POINT('Ctrl Pts',(-0.479780846242934,-0.992427501112665,
59.861775));
#41903=CARTESIAN_POINT('Ctrl Pts',(-0.437755592288797,-1.01443282934249,
59.861775));
#41904=CARTESIAN_POINT('Ctrl Pts',(-0.433388015774203,-1.01671978648681,
59.861775));
#41905=CARTESIAN_POINT('Ctrl Pts',(-0.429005145199489,-1.01897672231071,
59.861775));
#41906=CARTESIAN_POINT('Ctrl Pts',(-0.424607247138309,-1.02120342891482,
59.861775));
#41907=CARTESIAN_POINT('Ctrl Pts',(-0.382868534019858,-1.04233622163878,
59.861775));
#41908=CARTESIAN_POINT('Ctrl Pts',(-0.339778626521477,-1.06074970180182,
59.861775));
#41909=CARTESIAN_POINT('Ctrl Pts',(-0.29562133015478,-1.07641531260368,
59.861775));
#41910=CARTESIAN_POINT('Ctrl Pts',(-0.274591715400399,-1.08387595415473,
59.861775));
#41911=CARTESIAN_POINT('Ctrl Pts',(-0.253319595741797,-1.09071274018422,
59.861775));
#41912=CARTESIAN_POINT('Ctrl Pts',(-0.231833867236195,-1.09691905016394,
59.861775));
#41913=CARTESIAN_POINT('Ctrl Pts',(-0.220247415251091,-1.10026588164634,
59.861775));
#41914=CARTESIAN_POINT('Ctrl Pts',(-0.208598829633676,-1.10342932737445,
59.861775));
#41915=CARTESIAN_POINT('Ctrl Pts',(-0.19689255768268,-1.10640805572873,
59.861775));
#41916=CARTESIAN_POINT('Ctrl Pts',(-0.187496090203694,-1.10879904102506,
59.861775));
#41917=CARTESIAN_POINT('Ctrl Pts',(-0.178069361414857,-1.11106918282397,
59.861775));
#41918=CARTESIAN_POINT('Ctrl Pts',(-0.168622313084257,-1.11321671711805,
59.861775));
#41919=CARTESIAN_POINT('Ctrl Pts',(-0.121098578018619,-1.12401996986586,
59.861775));
#41920=CARTESIAN_POINT('Ctrl Pts',(-0.073005361777424,-1.13173889035925,
59.861775));
#41921=CARTESIAN_POINT('Ctrl Pts',(-0.0246593521685011,-1.13636033806869,
59.861775));
#41922=CARTESIAN_POINT('Ctrl Pts',(0.0230683985636239,-1.14092268573879,
59.861775));
#41923=CARTESIAN_POINT('Ctrl Pts',(0.0710436278401751,-1.1424664914666,
59.861775));
#41924=CARTESIAN_POINT('Ctrl Pts',(0.118980208527935,-1.14093288136104,
59.861775));
#41925=CARTESIAN_POINT('Ctrl Pts',(0.14321229178875,-1.14015763691861,59.861775));
#41926=CARTESIAN_POINT('Ctrl Pts',(0.167434691953048,-1.13859524577042,
59.861775));
#41927=CARTESIAN_POINT('Ctrl Pts',(0.191613851491352,-1.13625725196546,
59.861775));
#41928=CARTESIAN_POINT('Ctrl Pts',(0.207199962167851,-1.13475015945684,
59.861775));
#41929=CARTESIAN_POINT('Ctrl Pts',(0.222768107495521,-1.132920720623,59.861775));
#41930=CARTESIAN_POINT('Ctrl Pts',(0.238309236150123,-1.13077131215,59.861775));
#41931=CARTESIAN_POINT('Ctrl Pts',(0.247294863295863,-1.12952855922314,
59.861775));
#41932=CARTESIAN_POINT('Ctrl Pts',(0.256270239073691,-1.12817889864578,
59.861775));
#41933=CARTESIAN_POINT('Ctrl Pts',(0.265221037989145,-1.12672513730018,
59.861775));
#41934=CARTESIAN_POINT('Ctrl Pts',(0.313867380575837,-1.11882414732982,
59.861775));
#41935=CARTESIAN_POINT('Ctrl Pts',(0.361886766975759,-1.10783931741569,
59.861775));
#41936=CARTESIAN_POINT('Ctrl Pts',(0.409003407702753,-1.0939199257479,59.861775));
#41937=CARTESIAN_POINT('Ctrl Pts',(0.456548635540028,-1.07987391911436,
59.861775));
#41938=CARTESIAN_POINT('Ctrl Pts',(0.503175704622686,-1.06283956339786,
59.861775));
#41939=CARTESIAN_POINT('Ctrl Pts',(0.548601290212343,-1.04291756028592,
59.861775));
#41940=CARTESIAN_POINT('Ctrl Pts',(0.591117300761962,-1.02427159054261,
59.861775));
#41941=CARTESIAN_POINT('Ctrl Pts',(0.632581562956363,-1.0030954173452,59.861775));
#41942=CARTESIAN_POINT('Ctrl Pts',(0.672748867539255,-0.97943229058963,
59.861775));
#41943=CARTESIAN_POINT('',(-1.188225,-1.45515594291687E-16,59.861775));
#41944=CARTESIAN_POINT('Origin',(0.,0.,59.861775));
#41945=CARTESIAN_POINT('',(1.18460912750413,-0.0928893956975266,59.861775));
#41946=CARTESIAN_POINT('Origin',(0.,0.,59.861775));
#41947=CARTESIAN_POINT('Ctrl Pts',(1.18463057630127,-0.0928773270330193,
59.861775));
#41948=CARTESIAN_POINT('Ctrl Pts',(1.18495917433816,-0.0591973510751312,
59.861775));
#41949=CARTESIAN_POINT('Ctrl Pts',(1.18384723794147,-0.0255569108469606,
59.861775));
#41950=CARTESIAN_POINT('Ctrl Pts',(1.18127296688008,0.00795555060754574,
59.861775));
#41951=CARTESIAN_POINT('Ctrl Pts',(1.17757694805885,0.0560711861906696,
59.861775));
#41952=CARTESIAN_POINT('Ctrl Pts',(1.17086819176842,0.103924041630274,59.861775));
#41953=CARTESIAN_POINT('Ctrl Pts',(1.16122381979749,0.151244181532205,59.861775));
#41954=CARTESIAN_POINT('Ctrl Pts',(1.15737804746034,0.170113474999273,59.861775));
#41955=CARTESIAN_POINT('Ctrl Pts',(1.15306501652236,0.188897877747367,59.861775));
#41956=CARTESIAN_POINT('Ctrl Pts',(1.14828781990542,0.207579342678793,59.861775));
#41957=CARTESIAN_POINT('Ctrl Pts',(1.14557847714315,0.218174362281078,59.861775));
#41958=CARTESIAN_POINT('Ctrl Pts',(1.14272017734302,0.228734422458591,59.861775));
#41959=CARTESIAN_POINT('Ctrl Pts',(1.1397169789668,0.239245168892212,59.861775));
#41960=CARTESIAN_POINT('Ctrl Pts',(1.12618741947878,0.286596609364257,59.861775));
#41961=CARTESIAN_POINT('Ctrl Pts',(1.10970488146276,0.333012630300466,59.861775));
#41962=CARTESIAN_POINT('Ctrl Pts',(1.09035192020453,0.378202802308839,59.861775));
#41963=CARTESIAN_POINT('Ctrl Pts',(1.07747056795985,0.408281430373587,59.861775));
#41964=CARTESIAN_POINT('Ctrl Pts',(1.06331654234041,0.437816614433228,59.861775));
#41965=CARTESIAN_POINT('Ctrl Pts',(1.04790356112901,0.466715221191892,59.861775));
#41966=CARTESIAN_POINT('Ctrl Pts',(1.04254300086328,0.476766016751856,59.861775));
#41967=CARTESIAN_POINT('Ctrl Pts',(1.03703008545209,0.486739745783998,59.861775));
#41968=CARTESIAN_POINT('Ctrl Pts',(1.03136517466139,0.496632265600078,59.861775));
#41969=CARTESIAN_POINT('Ctrl Pts',(1.02625122763606,0.505562648470277,59.861775));
#41970=CARTESIAN_POINT('Ctrl Pts',(1.02101800912316,0.514418756608124,59.861775));
#41971=CARTESIAN_POINT('Ctrl Pts',(1.01566821899752,0.523194987724883,59.861775));
#41972=CARTESIAN_POINT('Ctrl Pts',(1.00990493839165,0.532649542277472,59.861775));
#41973=CARTESIAN_POINT('Ctrl Pts',(1.00400570856243,0.54201255557472,59.861775));
#41974=CARTESIAN_POINT('Ctrl Pts',(0.997971579640927,0.551280810079599,
59.861775));
#41975=CARTESIAN_POINT('Ctrl Pts',(0.971594934033771,0.591794605467841,
59.861775));
#41976=CARTESIAN_POINT('Ctrl Pts',(0.942643848491387,0.630500527183138,
59.861775));
#41977=CARTESIAN_POINT('Ctrl Pts',(0.911348678913813,0.667203480005342,
59.861775));
#41978=CARTESIAN_POINT('Ctrl Pts',(0.880279653768076,0.703641210797284,
59.861775));
#41979=CARTESIAN_POINT('Ctrl Pts',(0.846899360884351,0.738105471913161,
59.861775));
#41980=CARTESIAN_POINT('Ctrl Pts',(0.811401841668893,0.770365388497151,
59.861775));
#41981=CARTESIAN_POINT('Ctrl Pts',(0.792170102127397,0.787843069391074,
59.861775));
#41982=CARTESIAN_POINT('Ctrl Pts',(0.77231644980281,0.804672975392104,59.861775));
#41983=CARTESIAN_POINT('Ctrl Pts',(0.751869309712643,0.820812397933032,
59.861775));
#41984=CARTESIAN_POINT('Ctrl Pts',(0.744749793833871,0.826432004124786,
59.861775));
#41985=CARTESIAN_POINT('Ctrl Pts',(0.737558154141825,0.831967832124177,
59.861775));
#41986=CARTESIAN_POINT('Ctrl Pts',(0.730307446536889,0.83740945949028,59.861775));
#41987=CARTESIAN_POINT('Ctrl Pts',(0.692551663872584,0.865745024978379,
59.861775));
#41988=CARTESIAN_POINT('Ctrl Pts',(0.653119323526253,0.891591843549213,
59.861775));
#41989=CARTESIAN_POINT('Ctrl Pts',(0.612212142191562,0.914751484082298,
59.861775));
#41990=CARTESIAN_POINT('Ctrl Pts',(0.605291188285646,0.918669788873226,
59.861775));
#41991=CARTESIAN_POINT('Ctrl Pts',(0.59832796009732,0.922511069601298,59.861775));
#41992=CARTESIAN_POINT('Ctrl Pts',(0.591323369627692,0.926274231416198,
59.861775));
#41993=CARTESIAN_POINT('Ctrl Pts',(0.551834952455115,0.947489076777823,
59.861775));
#41994=CARTESIAN_POINT('Ctrl Pts',(0.511032589468169,0.966224558513573,
59.861775));
#41995=CARTESIAN_POINT('Ctrl Pts',(0.469164126081047,0.982399610517108,
59.861775));
#41996=CARTESIAN_POINT('Ctrl Pts',(0.449995116427187,0.989805177928087,
59.861775));
#41997=CARTESIAN_POINT('Ctrl Pts',(0.430602536035571,0.996673459296994,
59.861775));
#41998=CARTESIAN_POINT('Ctrl Pts',(0.41101004444375,1.00299367986045,59.861775));
#41999=CARTESIAN_POINT('Ctrl Pts',(0.396644935535153,1.00762763140739,59.861775));
#42000=CARTESIAN_POINT('Ctrl Pts',(0.382172358715336,1.01196692045316,59.861775));
#42001=CARTESIAN_POINT('Ctrl Pts',(0.367601731133845,1.01600663591634,59.861775));
#42002=CARTESIAN_POINT('Ctrl Pts',(0.359081682696219,1.01836882458859,59.861775));
#42003=CARTESIAN_POINT('Ctrl Pts',(0.350536793205264,1.0206261443741,59.861775));
#42004=CARTESIAN_POINT('Ctrl Pts',(0.341971425877663,1.02277764435025,59.861775));
#42005=CARTESIAN_POINT('Ctrl Pts',(0.297265461380135,1.03400715475785,59.861775));
#42006=CARTESIAN_POINT('Ctrl Pts',(0.251980969497039,1.04236390172438,59.861775));
#42007=CARTESIAN_POINT('Ctrl Pts',(0.206392409752112,1.04777705832953,59.861775));
#42008=CARTESIAN_POINT('Ctrl Pts',(0.162531617113603,1.05298506096674,59.861775));
#42009=CARTESIAN_POINT('Ctrl Pts',(0.118388411378249,1.05546820201981,59.861775));
#42010=CARTESIAN_POINT('Ctrl Pts',(0.0742092780586676,1.05511789517874,
59.861775));
#42011=CARTESIAN_POINT('Ctrl Pts',(0.0525758589890548,1.05494635866078,
59.861775));
#42012=CARTESIAN_POINT('Ctrl Pts',(0.0309339423407732,1.05409468861183,
59.861775));
#42013=CARTESIAN_POINT('Ctrl Pts',(0.00931474303316654,1.05256641039276,
59.861775));
#42014=CARTESIAN_POINT('Ctrl Pts',(-0.00776915395261585,1.0513587362653,
59.861775));
#42015=CARTESIAN_POINT('Ctrl Pts',(-0.0248388516191337,1.04972850975678,
59.861775));
#42016=CARTESIAN_POINT('Ctrl Pts',(-0.0418783779732828,1.04767648714608,
59.861775));
#42017=CARTESIAN_POINT('Ctrl Pts',(-0.0506706059106654,1.04661766366994,
59.861775));
#42018=CARTESIAN_POINT('Ctrl Pts',(-0.0594452838937768,1.04544765251369,
59.861775));
#42019=CARTESIAN_POINT('Ctrl Pts',(-0.0681982225184759,1.04416754258846,
59.861775));
#42020=CARTESIAN_POINT('Ctrl Pts',(-0.112958009502046,1.03762146132072,
59.861775));
#42021=CARTESIAN_POINT('Ctrl Pts',(-0.157169095981507,1.02819814056938,
59.861775));
#42022=CARTESIAN_POINT('Ctrl Pts',(-0.200557341352607,1.01597710620675,
59.861775));
#42023=CARTESIAN_POINT('Ctrl Pts',(-0.243177930293229,1.00397229528288,
59.861775));
#42024=CARTESIAN_POINT('Ctrl Pts',(-0.285005500695438,0.989267371338,59.861775));
#42025=CARTESIAN_POINT('Ctrl Pts',(-0.325758763954662,0.97189347978409,
59.861775));
#42026=CARTESIAN_POINT('Ctrl Pts',(-0.358468307116102,0.957948779158524,
59.861775));
#42027=CARTESIAN_POINT('Ctrl Pts',(-0.390485567095365,0.942283809933677,
59.861775));
#42028=CARTESIAN_POINT('Ctrl Pts',(-0.421648628688828,0.924896675066913,
59.861775));
#42029=CARTESIAN_POINT('Ctrl Pts',(-0.437855924241139,0.917335061595237,
55.9626150912667));
#42030=CARTESIAN_POINT('Ctrl Pts',(-0.59011828195518,0.844658263165578,
55.9705402130324));
#42031=CARTESIAN_POINT('Ctrl Pts',(-0.857585956829971,0.622054483027012,
55.9863904565638));
#42032=CARTESIAN_POINT('Ctrl Pts',(-1.05057757445303,0.136862273787097,
56.010165821861));
#42033=CARTESIAN_POINT('Ctrl Pts',(-0.988364686858664,-0.381513829574367,
56.0339411871581));
#42034=CARTESIAN_POINT('Ctrl Pts',(-0.686123743003436,-0.807263618083567,
56.0577165524553));
#42035=CARTESIAN_POINT('Ctrl Pts',(-0.217232371214364,-1.03693712275359,
56.0814919177525));
#42036=CARTESIAN_POINT('Ctrl Pts',(0.304414618904077,-1.01477332192588,
56.1052672830496));
#42037=CARTESIAN_POINT('Ctrl Pts',(0.752129524692829,-0.746145432160931,
56.1290426483468));
#42038=CARTESIAN_POINT('Ctrl Pts',(1.01717154895307,-0.296300389836015,
56.1528180136439));
#42039=CARTESIAN_POINT('Ctrl Pts',(1.03517049480264,0.225508677645759,56.1765933789411));
#42040=CARTESIAN_POINT('Ctrl Pts',(0.801754274033107,0.69254746844306,56.2003687442382));
#42041=CARTESIAN_POINT('Ctrl Pts',(0.373613677358384,0.991385317760177,
56.2241441095354));
#42042=CARTESIAN_POINT('Ctrl Pts',(-0.14526763822163,1.04944237138876,56.2479194748325));
#42043=CARTESIAN_POINT('Ctrl Pts',(-0.628867346267627,0.852618234981034,
56.2716948401297));
#42044=CARTESIAN_POINT('Ctrl Pts',(-0.959732162422036,0.448716132860876,
56.2954702054268));
#42045=CARTESIAN_POINT('Ctrl Pts',(-1.0575039415156,-0.0641669975384679,
56.319245570724));
#42046=CARTESIAN_POINT('Ctrl Pts',(-0.898436564193858,-0.561465699584117,
56.3430209360212));
#42047=CARTESIAN_POINT('Ctrl Pts',(-0.521163199217816,-0.922399539433787,
56.3667963013183));
#42048=CARTESIAN_POINT('Ctrl Pts',(-0.0173133632032956,-1.05930743344434,
56.3905716666155));
#42049=CARTESIAN_POINT('Ctrl Pts',(0.49074142153069,-0.938938149241069,
56.4143470319126));
#42050=CARTESIAN_POINT('Ctrl Pts',(0.879608363221454,-0.590526136845567,
56.4381223972097));
#42051=CARTESIAN_POINT('Ctrl Pts',(1.05484217994403,-0.0986912679291979,
56.4618977625069));
#42052=CARTESIAN_POINT('Ctrl Pts',(0.973883308267136,0.417113045610174,
56.4856731278041));
#42053=CARTESIAN_POINT('Ctrl Pts',(0.656394472537722,0.831611861009717,
56.5094484931012));
#42054=CARTESIAN_POINT('Ctrl Pts',(0.179485139828959,1.0441346060376,56.5332238583984));
#42055=CARTESIAN_POINT('Ctrl Pts',(-0.341016287857761,1.00306524332296,
56.5569992236956));
#42056=CARTESIAN_POINT('Ctrl Pts',(-0.778694065497443,0.718378412332483,
56.5807745889927));
#42057=CARTESIAN_POINT('Ctrl Pts',(-1.02724807670217,0.259216858745684,
56.6045499542899));
#42058=CARTESIAN_POINT('Ctrl Pts',(-1.02631126225859,-0.262901471862694,
56.628325319587));
#42059=CARTESIAN_POINT('Ctrl Pts',(-0.776111149103991,-0.721168132395479,
56.6521006848841));
#42060=CARTESIAN_POINT('Ctrl Pts',(-0.337414590176968,-1.00428252264095,
56.6758760501813));
#42061=CARTESIAN_POINT('Ctrl Pts',(0.18323086366488,-1.043483800328,56.6996514154785));
#42062=CARTESIAN_POINT('Ctrl Pts',(0.659374487328757,-0.82925103340682,
56.7234267807756));
#42063=CARTESIAN_POINT('Ctrl Pts',(0.975373848875025,-0.41361557741103,
56.7472021460728));
#42064=CARTESIAN_POINT('Ctrl Pts',(1.05448123428539,0.102475936132846,56.77097751137));
#42065=CARTESIAN_POINT('Ctrl Pts',(0.877483595272346,0.593678811289621,
56.7947528766671));
#42066=CARTESIAN_POINT('Ctrl Pts',(0.48736888002166,0.940693130480272,56.8185282419642));
#42067=CARTESIAN_POINT('Ctrl Pts',(-0.02111457889448,1.0592384837724,56.8423036072614));
#42068=CARTESIAN_POINT('Ctrl Pts',(-0.524469876618518,0.920523405170176,
56.8660789725585));
#42069=CARTESIAN_POINT('Ctrl Pts',(-0.900445600203663,0.558238042433696,
56.8898543378557));
#42070=CARTESIAN_POINT('Ctrl Pts',(-1.05772739644889,0.0603717297067289,
56.9136297031529));
#42071=CARTESIAN_POINT('Ctrl Pts',(-0.958115763116474,-0.452157246335915,
56.93740506845));
#42072=CARTESIAN_POINT('Ctrl Pts',(-0.62580367676965,-0.854869433941773,
56.9611804337472));
#42073=CARTESIAN_POINT('Ctrl Pts',(-0.141500771893025,-1.04995691459222,
56.9849557990443));
#42074=CARTESIAN_POINT('Ctrl Pts',(0.377168850439841,-0.990038205931583,
57.0087311643415));
#42075=CARTESIAN_POINT('Ctrl Pts',(0.804234341269022,-0.689665944693458,
57.0325065296386));
#42076=CARTESIAN_POINT('Ctrl Pts',(1.0359730221788,-0.221792444109516,57.0562818949358));
#42077=CARTESIAN_POINT('Ctrl Pts',(1.01610182372747,0.29994845351169,57.0800572602329));
#42078=CARTESIAN_POINT('Ctrl Pts',(0.749446923564514,0.748839969356621,
57.1038326255301));
#42079=CARTESIAN_POINT('Ctrl Pts',(0.300771598169799,1.0158584727612,57.1276079908272));
#42080=CARTESIAN_POINT('Ctrl Pts',(-0.220953028616557,1.03615237783422,
57.1513833561244));
#42081=CARTESIAN_POINT('Ctrl Pts',(-0.689014129727543,0.804792842899423,
57.1751587214215));
#42082=CARTESIAN_POINT('Ctrl Pts',(-0.989732299751159,0.377970853076824,
57.1989340867187));
#42083=CARTESIAN_POINT('Ctrl Pts',(-1.05007121355009,-0.140650053038654,
57.2227094520158));
#42084=CARTESIAN_POINT('Ctrl Pts',(-0.855376177906754,-0.62511085834112,
57.246484817313));
#42085=CARTESIAN_POINT('Ctrl Pts',(-0.452933360879266,-0.957749112006351,
57.2702601826102));
#42086=CARTESIAN_POINT('Ctrl Pts',(0.0595147418551541,-1.0577759623135,
57.2940355479073));
#42087=CARTESIAN_POINT('Ctrl Pts',(0.557508320487304,-0.900897587705596,
57.3178109132045));
#42088=CARTESIAN_POINT('Ctrl Pts',(0.920098178889751,-0.525215510195677,
57.3415862785016));
#42089=CARTESIAN_POINT('Ctrl Pts',(1.0592210291418,-0.0219727642805258,
57.3653616437988));
#42090=CARTESIAN_POINT('Ctrl Pts',(0.941087686758059,0.486606572888925,
57.3891370090959));
#42091=CARTESIAN_POINT('Ctrl Pts',(0.594389551407591,0.877002310215783,
57.4129123743931));
#42092=CARTESIAN_POINT('Ctrl Pts',(0.103330240503893,1.05439786245219,57.4366877396903));
#42093=CARTESIAN_POINT('Ctrl Pts',(-0.412825196255343,0.975708639032718,
57.4604631049874));
#42094=CARTESIAN_POINT('Ctrl Pts',(-0.828716537711619,0.660046127986225,
57.4842384702846));
#42095=CARTESIAN_POINT('Ctrl Pts',(-1.04333500466809,0.18407623143842,57.5080138355817));
#42096=CARTESIAN_POINT('Ctrl Pts',(-1.00455556546515,-0.336600812297502,
57.5317892008789));
#42097=CARTESIAN_POINT('Ctrl Pts',(-0.721796698973036,-0.775526605796326,
57.555564566176));
#42098=CARTESIAN_POINT('Ctrl Pts',(-0.263732900340999,-1.02609792331145,
57.5793399314732));
#42099=CARTESIAN_POINT('Ctrl Pts',(0.258384499898145,-1.02745775638647,
57.6031152967703));
#42100=CARTESIAN_POINT('Ctrl Pts',(0.717747280609244,-0.779275838278319,
57.6268906620675));
#42101=CARTESIAN_POINT('Ctrl Pts',(1.00278862358054,-0.341828856833032,
57.6506660273646));
#42102=CARTESIAN_POINT('Ctrl Pts',(1.04427968174507,0.178639125727723,57.6744413926618));
#42103=CARTESIAN_POINT('Ctrl Pts',(0.832143397191218,0.655720487294243,
57.6982167579589));
#42104=CARTESIAN_POINT('Ctrl Pts',(0.417901946483455,0.973545044706037,
57.7219921232561));
#42105=CARTESIAN_POINT('Ctrl Pts',(-0.0978366051027944,1.05492179314312,
57.7457674885532));
#42106=CARTESIAN_POINT('Ctrl Pts',(-0.589813286563081,0.880086517303837,
57.7695428538504));
#42107=CARTESIAN_POINT('Ctrl Pts',(-0.93854024365738,0.491501985735445,
57.7933182191476));
#42108=CARTESIAN_POINT('Ctrl Pts',(-1.05932111294186,-0.0164551092965639,
57.8170935844447));
#42109=CARTESIAN_POINT('Ctrl Pts',(-0.922821481937435,-0.520415702512074,
57.8408689497419));
#42110=CARTESIAN_POINT('Ctrl Pts',(-0.562193425992196,-0.897981371030322,
57.864644315039));
#42111=CARTESIAN_POINT('Ctrl Pts',(-0.0650237641719233,-1.05745160694911,
57.8884196803362));
#42112=CARTESIAN_POINT('Ctrl Pts',(0.447938414546611,-0.960095395114365,
57.9121950456334));
#42113=CARTESIAN_POINT('Ctrl Pts',(0.852108445175959,-0.629557931096218,
57.9359704109305));
#42114=CARTESIAN_POINT('Ctrl Pts',(1.04932433848386,-0.146117841524369,
57.9597457762276));
#42115=CARTESIAN_POINT('Ctrl Pts',(0.991687678140017,0.372810327072094,
57.9835211415248));
#42116=CARTESIAN_POINT('Ctrl Pts',(0.693196852949359,0.80119293182569,58.007296506822));
#42117=CARTESIAN_POINT('Ctrl Pts',(0.226347226119961,1.03498740290602,58.0310718721191));
#42118=CARTESIAN_POINT('Ctrl Pts',(-0.295476031333513,1.01741137493825,
58.0548472374163));
#42119=CARTESIAN_POINT('Ctrl Pts',(-0.745536137617694,0.752733590623157,
58.0786226027134));
#42120=CARTESIAN_POINT('Ctrl Pts',(-1.01452564299876,0.305237138376526,
58.1023979680106));
#42121=CARTESIAN_POINT('Ctrl Pts',(-1.03711425841572,-0.216393174423657,
58.1261733333077));
#42122=CARTESIAN_POINT('Ctrl Pts',(-0.807815818999105,-0.685467427031471,
58.1499486986049));
#42123=CARTESIAN_POINT('Ctrl Pts',(-0.382320725410081,-0.988060146887956,
58.173724063902));
#42124=CARTESIAN_POINT('Ctrl Pts',(0.136029751029905,-1.05067973130782,
58.1974994291992));
#42125=CARTESIAN_POINT('Ctrl Pts',(0.62134227328246,-0.858117573749964,
58.2212747944964));
#42126=CARTESIAN_POINT('Ctrl Pts',(0.955747531469626,-0.457141823765944,
58.2450501597935));
#42127=CARTESIAN_POINT('Ctrl Pts',(1.05802751617526,0.0548613339460823,
58.2688255250907));
#42128=CARTESIAN_POINT('Ctrl Pts',(0.903341180323916,0.553540154710871,
58.2926008903878));
#42129=CARTESIAN_POINT('Ctrl Pts',(0.5292576588922,0.917779015586153,58.316376255685));
#42130=CARTESIAN_POINT('Ctrl Pts',(0.0266317402610465,1.05911413046801,
58.3401516209821));
#42131=CARTESIAN_POINT('Ctrl Pts',(-0.482462309113668,0.94321901551604,
58.3639269862793));
#42132=CARTESIAN_POINT('Ctrl Pts',(-0.874379288435858,0.598241465380611,
58.3877023515764));
#42133=CARTESIAN_POINT('Ctrl Pts',(-1.05393314384533,0.107967213776402,
58.4114777168736));
#42134=CARTESIAN_POINT('Ctrl Pts',(-0.977515091202718,-0.408529359308828,
58.4352530821707));
#42135=CARTESIAN_POINT('Ctrl Pts',(-0.66368501246902,-0.825805179912512,
58.4590284474679));
#42136=CARTESIAN_POINT('Ctrl Pts',(-0.188663761430564,-1.0425152162291,
58.482803812765));
#42137=CARTESIAN_POINT('Ctrl Pts',(0.33217882398349,-1.00602645086662,58.5065791780622));
#42138=CARTESIAN_POINT('Ctrl Pts',(0.772344140743365,-0.725201019859825,
58.5303545433593));
#42139=CARTESIAN_POINT('Ctrl Pts',(1.02492791636524,-0.268243839074722,
58.5541299086565));
#42140=CARTESIAN_POINT('Ctrl Pts',(1.02858437064807,0.253862528556006,58.5779052739536));
#42141=CARTESIAN_POINT('Ctrl Pts',(0.782425449558309,0.714312541419944,
58.6016806392508));
#42142=CARTESIAN_POINT('Ctrl Pts',(0.346236509580231,1.00127532196696,58.625456004548));
#42143=CARTESIAN_POINT('Ctrl Pts',(-0.174043931374068,1.04505535781517,
58.6492313698451));
#42144=CARTESIAN_POINT('Ctrl Pts',(-0.652053799988115,0.83501966016819,
58.6730067351423));
#42145=CARTESIAN_POINT('Ctrl Pts',(-0.97169740380609,0.422180229739439,
58.6967821004394));
#42146=CARTESIAN_POINT('Ctrl Pts',(-1.05534194074397,-0.0931953810716716,
58.7205574657366));
#42147=CARTESIAN_POINT('Ctrl Pts',(-0.882672410895779,-0.585936349776809,
58.7443328310337));
#42148=CARTESIAN_POINT('Ctrl Pts',(-0.495625581575281,-0.936369197397321,
58.7681081963309));
#42149=CARTESIAN_POINT('Ctrl Pts',(0.0117953213153582,-1.05938324573377,
58.7918835616281));
#42150=CARTESIAN_POINT('Ctrl Pts',(0.516351459091809,-0.925101703403523,
58.8156589269252));
#42151=CARTESIAN_POINT('Ctrl Pts',(0.895499767177114,-0.566137931896525,
58.8394342922223));
#42152=CARTESIAN_POINT('Ctrl Pts',(1.05715535724409,-0.0696745405184991,
58.8632096575195));
#42153=CARTESIAN_POINT('Ctrl Pts',(0.962056450613156,0.443710915777326,
58.8869850228166));
#42154=CARTESIAN_POINT('Ctrl Pts',(0.633300004359957,0.84933096930703,58.9107603881138));
#42155=CARTESIAN_POINT('Ctrl Pts',(0.150732083980457,1.04867145942151,58.934535753411));
#42156=CARTESIAN_POINT('Ctrl Pts',(-0.368444590347487,0.993317962582985,
58.9583111187081));
#42157=CARTESIAN_POINT('Ctrl Pts',(-0.798136020423016,0.696714348818546,
58.9820864840053));
#42158=CARTESIAN_POINT('Ctrl Pts',(-1.03398175807884,0.230897628629093,
59.0058618493024));
#42159=CARTESIAN_POINT('Ctrl Pts',(-1.01870124066612,-0.290997892108609,
59.0296372145996));
#42160=CARTESIAN_POINT('Ctrl Pts',(-0.756005693342733,-0.742217880800317,
59.0534125798968));
#42161=CARTESIAN_POINT('Ctrl Pts',(-0.3096967726728,-1.01317318358827,59.0771879451939));
#42162=CARTESIAN_POINT('Ctrl Pts',(0.211829133326388,-1.03805607229115,
59.1009633104911));
#42163=CARTESIAN_POINT('Ctrl Pts',(0.681907461502236,-0.810823164995865,
59.1247386757882));
#42164=CARTESIAN_POINT('Ctrl Pts',(0.986368876446939,-0.386663200373609,
59.1485140410854));
#42165=CARTESIAN_POINT('Ctrl Pts',(1.0512679198866,0.131406817036291,59.1722894063825));
#42166=CARTESIAN_POINT('Ctrl Pts',(0.860842366221901,0.617561666122401,
59.1960647716797));
#42167=CARTESIAN_POINT('Ctrl Pts',(0.461341441599518,0.953727458558869,
59.2198401369768));
#42168=CARTESIAN_POINT('Ctrl Pts',(-0.0502068645469796,1.05825859868873,
59.243615502274));
#42169=CARTESIAN_POINT('Ctrl Pts',(-0.549561278709315,0.905767294557619,
59.2673908675711));
#42170=CARTESIAN_POINT('Ctrl Pts',(-0.91544209454521,0.533289567195347,
59.2911662328683));
#42171=CARTESIAN_POINT('Ctrl Pts',(-1.05898673942326,0.0312902009549694,
59.3149415981654));
#42172=CARTESIAN_POINT('Ctrl Pts',(-0.945332094305355,-0.478308710369975,
59.3387169634626));
#42173=CARTESIAN_POINT('Ctrl Pts',(-0.602081804228732,-0.871739348642251,
59.3624923287598));
#42174=CARTESIAN_POINT('Ctrl Pts',(-0.112602098016971,-1.05344803311272,
59.3862676940569));
#42175=CARTESIAN_POINT('Ctrl Pts',(0.404225617853905,-0.979302629822281,
59.4100430593541));
#42176=CARTESIAN_POINT('Ctrl Pts',(0.822877844024298,-0.667311055587846,
59.4338184246512));
#42177=CARTESIAN_POINT('Ctrl Pts',(1.04167525640482,-0.193247641021974,
59.4575937899483));
#42178=CARTESIAN_POINT('Ctrl Pts',(1.00747787145168,0.327750408428632,59.4813691552455));
#42179=CARTESIAN_POINT('Ctrl Pts',(0.728591308296158,0.769146732015046,
59.5051445205427));
#42180=CARTESIAN_POINT('Ctrl Pts',(0.272749589451039,1.02373807828526,59.5289198858398));
#42181=CARTESIAN_POINT('Ctrl Pts',(-0.24933564917612,1.02969108371093,59.552695251137));
#42182=CARTESIAN_POINT('Ctrl Pts',(-0.710863972995126,0.785559920997844,
59.5764706164341));
#42183=CARTESIAN_POINT('Ctrl Pts',(-0.999742664943908,0.350637465297931,
59.6002459817313));
#42184=CARTESIAN_POINT('Ctrl Pts',(-1.04581077501601,-0.169445374199638,
59.6240213470285));
#42185=CARTESIAN_POINT('Ctrl Pts',(-0.837879849628336,-0.648374486381346,
59.6477967123256));
#42186=CARTESIAN_POINT('Ctrl Pts',(-0.426450165346835,-0.969830983982369,
59.6715720776227));
#42187=CARTESIAN_POINT('Ctrl Pts',(0.0885519692748135,-1.0557416239719,
59.6953474429199));
#42188=CARTESIAN_POINT('Ctrl Pts',(0.582048910852398,-0.885241334592178,
59.7191228082171));
#42189=CARTESIAN_POINT('Ctrl Pts',(0.93417826195316,-0.499739406633171,
59.7428981735142));
#42190=CARTESIAN_POINT('Ctrl Pts',(1.05942882546267,0.00713467400835743,
59.7666735388114));
#42191=CARTESIAN_POINT('Ctrl Pts',(0.927356096326115,0.51227749022626,59.7904489041085));
#42192=CARTESIAN_POINT('Ctrl Pts',(0.570091202696139,0.892995264566529,
59.8142242694056));
#42193=CARTESIAN_POINT('Ctrl Pts',(0.0742928706965789,1.05682828433461,
59.8379996347028));
#42194=CARTESIAN_POINT('Ctrl Pts',(-0.268131168947707,0.994883332089929,
59.8538498782343));
#42195=CARTESIAN_POINT('Ctrl Pts',(-0.421648628688828,0.924896675066913,
59.861775));
#42196=CARTESIAN_POINT('Ctrl Pts',(-0.462516886549903,0.969001292713887,
55.9956683941778));
#42197=CARTESIAN_POINT('Ctrl Pts',(-0.623354979013081,0.892231184847107,
56.0035935159435));
#42198=CARTESIAN_POINT('Ctrl Pts',(-0.905886993282922,0.657089893788024,
56.0194437594749));
#42199=CARTESIAN_POINT('Ctrl Pts',(-1.10974830284028,0.144570643569252,
56.0432191247721));
#42200=CARTESIAN_POINT('Ctrl Pts',(-1.04403145517334,-0.403001487158792,
56.0669944900692));
#42201=CARTESIAN_POINT('Ctrl Pts',(-0.72476766861592,-0.85273039506803,
56.0907698553664));
#42202=CARTESIAN_POINT('Ctrl Pts',(-0.22946735313918,-1.09533959234472,
56.1145452206636));
#42203=CARTESIAN_POINT('Ctrl Pts',(0.321559887535626,-1.07192747985427,
56.1383205859607));
#42204=CARTESIAN_POINT('Ctrl Pts',(0.79449103411378,-0.788169904962737,
56.1620959512579));
#42205=CARTESIAN_POINT('Ctrl Pts',(1.07446078004833,-0.312988648099244,
56.185871316555));
#42206=CARTESIAN_POINT('Ctrl Pts',(1.09347346420912,0.238209798475307,56.2096466818521));
#42207=CARTESIAN_POINT('Ctrl Pts',(0.846910753226789,0.731553191720428,
56.2334220471493));
#42208=CARTESIAN_POINT('Ctrl Pts',(0.39465638183097,1.04722221433094,56.2571974124465));
#42209=CARTESIAN_POINT('Ctrl Pts',(-0.153449415725439,1.10854916276288,
56.2809727777436));
#42210=CARTESIAN_POINT('Ctrl Pts',(-0.664286471749138,0.900639478939484,
56.3047481430408));
#42211=CARTESIAN_POINT('Ctrl Pts',(-1.01378628701798,0.473988764855061,
56.328523508338));
#42212=CARTESIAN_POINT('Ctrl Pts',(-1.11706477739624,-0.0677810171740453,
56.3522988736351));
#42213=CARTESIAN_POINT('Ctrl Pts',(-0.949038392374679,-0.593088623218428,
56.3760742389323));
#42214=CARTESIAN_POINT('Ctrl Pts',(-0.550516201657841,-0.974351012546832,
56.3998496042294));
#42215=CARTESIAN_POINT('Ctrl Pts',(-0.0182884880645982,-1.11896984576603,
56.4236249695266));
#42216=CARTESIAN_POINT('Ctrl Pts',(0.518381005763089,-0.991821111482199,
56.4474003348237));
#42217=CARTESIAN_POINT('Ctrl Pts',(0.929149747706489,-0.623785805144751,
56.4711757001208));
#42218=CARTESIAN_POINT('Ctrl Pts',(1.11425309984053,-0.104249766750074,
56.494951065418));
#42219=CARTESIAN_POINT('Ctrl Pts',(1.02873445502263,0.44060572556903,56.5187264307152));
#42220=CARTESIAN_POINT('Ctrl Pts',(0.693363983399069,0.878449982009057,
56.5425017960123));
#42221=CARTESIAN_POINT('Ctrl Pts',(0.189594118657963,1.10294245295529,56.5662771613095));
#42222=CARTESIAN_POINT('Ctrl Pts',(-0.360223039110721,1.05955997775346,
56.5900525266066));
#42223=CARTESIAN_POINT('Ctrl Pts',(-0.822551745469627,0.758838988447034,
56.6138278919038));
#42224=CARTESIAN_POINT('Ctrl Pts',(-1.08510483893557,0.273816494903183,
56.637603257201));
#42225=CARTESIAN_POINT('Ctrl Pts',(-1.08411526114131,-0.277708633144708,
56.6613786224981));
#42226=CARTESIAN_POINT('Ctrl Pts',(-0.819823353817542,-0.761785831384277,
56.6851539877952));
#42227=CARTESIAN_POINT('Ctrl Pts',(-0.356418486276366,-1.06084581679102,
56.7089293530924));
#42228=CARTESIAN_POINT('Ctrl Pts',(0.193550809502023,-1.10225499250565,
56.7327047183896));
#42229=CARTESIAN_POINT('Ctrl Pts',(0.696511838861817,-0.875956187653155,
56.7564800836867));
#42230=CARTESIAN_POINT('Ctrl Pts',(1.03030894599802,-0.436911272638936,
56.7802554489839));
#42231=CARTESIAN_POINT('Ctrl Pts',(1.11387182496675,0.108247595390182,56.804030814281));
#42232=CARTESIAN_POINT('Ctrl Pts',(0.926905308378269,0.62711604481364,56.8278061795782));
#42233=CARTESIAN_POINT('Ctrl Pts',(0.514818515655831,0.99367493693886,56.8515815448753));
#42234=CARTESIAN_POINT('Ctrl Pts',(-0.0223037961813828,1.11889701270422,
56.8753569101725));
#42235=CARTESIAN_POINT('Ctrl Pts',(-0.554009118052303,0.972369210473793,
56.8991322754696));
#42236=CARTESIAN_POINT('Ctrl Pts',(-0.951160581498487,0.589679177660173,
56.9229076407668));
#42237=CARTESIAN_POINT('Ctrl Pts',(-1.11730081777918,0.0637719919126017,
56.946683006064));
#42238=CARTESIAN_POINT('Ctrl Pts',(-1.01207884871958,-0.47762368904501,
56.9704583713611));
#42239=CARTESIAN_POINT('Ctrl Pts',(-0.66105024997122,-0.903017470138595,
56.9942337366583));
#42240=CARTESIAN_POINT('Ctrl Pts',(-0.149470391599245,-1.10909268611676,
57.0180091019554));
#42241=CARTESIAN_POINT('Ctrl Pts',(0.398411789703155,-1.04579923034397,
57.0417844672526));
#42242=CARTESIAN_POINT('Ctrl Pts',(0.849530503041471,-0.728509374520757,
57.0655598325497));
#42243=CARTESIAN_POINT('Ctrl Pts',(1.0943211916072,-0.234284258886341,57.0893351978469));
#42244=CARTESIAN_POINT('Ctrl Pts',(1.07333080565855,0.316842178358381,57.113110563144));
#42245=CARTESIAN_POINT('Ctrl Pts',(0.791657343273874,0.791016204134322,
57.1368859284412));
#42246=CARTESIAN_POINT('Ctrl Pts',(0.317711684246903,1.07307374865641,57.1606612937383));
#42247=CARTESIAN_POINT('Ctrl Pts',(-0.233397565755486,1.09451064894862,
57.1844366590355));
#42248=CARTESIAN_POINT('Ctrl Pts',(-0.727820847971375,0.850120460652928,
57.2082120243326));
#42249=CARTESIAN_POINT('Ctrl Pts',(-1.04547609488705,0.399258962807661,
57.2319873896298));
#42250=CARTESIAN_POINT('Ctrl Pts',(-1.10921342263122,-0.148571758478,57.255762754927));
#42251=CARTESIAN_POINT('Ctrl Pts',(-0.903552754984561,-0.660318410558366,
57.2795381202241));
#42252=CARTESIAN_POINT('Ctrl Pts',(-0.478443515984253,-1.01169154705135,
57.3033134855213));
#42253=CARTESIAN_POINT('Ctrl Pts',(0.0628667367111055,-1.11735211897495,
57.3270888508185));
#42254=CARTESIAN_POINT('Ctrl Pts',(0.588908356246074,-0.951638025882776,
57.3508642161155));
#42255=CARTESIAN_POINT('Ctrl Pts',(0.971920034559035,-0.554796747273525,
57.3746395814127));
#42256=CARTESIAN_POINT('Ctrl Pts',(1.11887857499228,-0.0232103163649987,
57.3984149467099));
#42257=CARTESIAN_POINT('Ctrl Pts',(0.994091715452223,0.514013273789476,
57.4221903120071));
#42258=CARTESIAN_POINT('Ctrl Pts',(0.627866815303003,0.926396916339742,
57.4459656773042));
#42259=CARTESIAN_POINT('Ctrl Pts',(0.10915001597191,1.11378375745737,57.4697410426014));
#42260=CARTESIAN_POINT('Ctrl Pts',(-0.436076375561883,1.03066259223828,
57.4935164078985));
#42261=CARTESIAN_POINT('Ctrl Pts',(-0.875391588041422,0.697221307727207,
57.5172917731957));
#42262=CARTESIAN_POINT('Ctrl Pts',(-1.10209781636267,0.194443790158363,
57.5410671384928));
#42263=CARTESIAN_POINT('Ctrl Pts',(-1.0611342379587,-0.355558874723069,
57.56484250379));
#42264=CARTESIAN_POINT('Ctrl Pts',(-0.762449800147398,-0.819205887807036,
57.5886178690872));
#42265=CARTESIAN_POINT('Ctrl Pts',(-0.278586889415522,-1.08388990649803,
57.6123932343843));
#42266=CARTESIAN_POINT('Ctrl Pts',(0.272937255862792,-1.08532632821866,
57.6361685996814));
#42267=CARTESIAN_POINT('Ctrl Pts',(0.758172310063855,-0.823166284911474,
57.6599439649786));
#42268=CARTESIAN_POINT('Ctrl Pts',(1.05926777820804,-0.361081373671809,
57.6837193302757));
#42269=CARTESIAN_POINT('Ctrl Pts',(1.10309569963031,0.188700455271399,57.7074946955729));
#42270=CARTESIAN_POINT('Ctrl Pts',(0.879011455421081,0.692652037895677,
57.7312700608701));
#42271=CARTESIAN_POINT('Ctrl Pts',(0.441439058991073,1.02837713974961,57.7550454261672));
#42272=CARTESIAN_POINT('Ctrl Pts',(-0.103346967524035,1.11433719702167,
57.7788207914643));
#42273=CARTESIAN_POINT('Ctrl Pts',(-0.623032805641989,0.929654832427817,
57.8025961567615));
#42274=CARTESIAN_POINT('Ctrl Pts',(-0.991400795023013,0.519184406536112,
57.8263715220587));
#42275=CARTESIAN_POINT('Ctrl Pts',(-1.11898429572149,-0.0173818955010686,
57.8501468873558));
#42276=CARTESIAN_POINT('Ctrl Pts',(-0.97479671973563,-0.549726604372732,
57.873922252653));
#42277=CARTESIAN_POINT('Ctrl Pts',(-0.59385733670132,-0.948557561779218,
57.8976976179501));
#42278=CARTESIAN_POINT('Ctrl Pts',(-0.0686860386979539,-1.1170094952374,
57.9214729832473));
#42279=CARTESIAN_POINT('Ctrl Pts',(0.473167243817168,-1.01416997773597,
57.9452483485444));
#42280=CARTESIAN_POINT('Ctrl Pts',(0.900100976705333,-0.665015951761027,
57.9690237138416));
#42281=CARTESIAN_POINT('Ctrl Pts',(1.10842448199767,-0.154347504258106,
57.9927990791387));
#42282=CARTESIAN_POINT('Ctrl Pts',(1.04754160428037,0.393807785174727,58.0165744444359));
#42283=CARTESIAN_POINT('Ctrl Pts',(0.73223915092162,0.84631779505107,58.040349809733));
#42284=CARTESIAN_POINT('Ctrl Pts',(0.239095575755094,1.09328006019357,58.0641251750302));
#42285=CARTESIAN_POINT('Ctrl Pts',(-0.31211786000007,1.07471411353508,58.0879005403274));
#42286=CARTESIAN_POINT('Ctrl Pts',(-0.787526293675256,0.795129122301928,
58.1116759056246));
#42287=CARTESIAN_POINT('Ctrl Pts',(-1.07166585113145,0.322428733026724,
58.1354512709217));
#42288=CARTESIAN_POINT('Ctrl Pts',(-1.09552670465818,-0.228580891028345,
58.1592266362188));
#42289=CARTESIAN_POINT('Ctrl Pts',(-0.853313697095174,-0.724074387554404,
58.1830020015159));
#42290=CARTESIAN_POINT('Ctrl Pts',(-0.403853829057226,-1.04370976287392,
58.2067773668132));
#42291=CARTESIAN_POINT('Ctrl Pts',(0.143691231387472,-1.10985621338301,
58.2305527321103));
#42292=CARTESIAN_POINT('Ctrl Pts',(0.656337570899634,-0.906448551980799,
58.2543280974075));
#42293=CARTESIAN_POINT('Ctrl Pts',(1.00957723330847,-0.482889008311166,
58.2781034627046));
#42294=CARTESIAN_POINT('Ctrl Pts',(1.11761784087684,0.0579512391266419,
58.3018788280018));
#42295=CARTESIAN_POINT('Ctrl Pts',(0.954219246753043,0.584716695065718,
58.3256541932989));
#42296=CARTESIAN_POINT('Ctrl Pts',(0.559066558246913,0.969470251122989,
58.3494295585961));
#42297=CARTESIAN_POINT('Ctrl Pts',(0.0281316956263525,1.11876565556139,
58.3732049238932));
#42298=CARTESIAN_POINT('Ctrl Pts',(-0.509635596402341,0.99634308510781,
58.3969802891904));
#42299=CARTESIAN_POINT('Ctrl Pts',(-0.923626160481851,0.631935677135001,
58.4207556544875));
#42300=CARTESIAN_POINT('Ctrl Pts',(-1.11329286492568,0.114048153286674,
58.4445310197847));
#42301=CARTESIAN_POINT('Ctrl Pts',(-1.03257078757632,-0.431538588085164,
58.4683063850818));
#42302=CARTESIAN_POINT('Ctrl Pts',(-0.701065141802112,-0.872316256476116,
58.492081750379));
#42303=CARTESIAN_POINT('Ctrl Pts',(-0.199289699443702,-1.10123185572256,
58.5158571156762));
#42304=CARTESIAN_POINT('Ctrl Pts',(0.350887830769737,-1.06268796670529,
58.5396324809733));
#42305=CARTESIAN_POINT('Ctrl Pts',(0.815844179659772,-0.766045859513509,
58.5634078462705));
#42306=CARTESIAN_POINT('Ctrl Pts',(1.08265400231119,-0.283351893662422,
58.5871832115676));
#42307=CARTESIAN_POINT('Ctrl Pts',(1.08651639575406,0.268160597627874,58.6109585768647));
#42308=CARTESIAN_POINT('Ctrl Pts',(0.826493288892493,0.754544119172755,
58.6347339421619));
#42309=CARTESIAN_POINT('Ctrl Pts',(0.365737274649193,1.05766924427947,58.6585093074591));
#42310=CARTESIAN_POINT('Ctrl Pts',(-0.183846449951664,1.10391506340057,
58.6822846727562));
#42311=CARTESIAN_POINT('Ctrl Pts',(-0.688778835084223,0.882049715550399,
58.7060600380533));
#42312=CARTESIAN_POINT('Ctrl Pts',(-1.02642543584613,0.445958304116661,
58.7298354033505));
#42313=CARTESIAN_POINT('Ctrl Pts',(-1.11478100821498,-0.098444340039033,
58.7536107686477));
#42314=CARTESIAN_POINT('Ctrl Pts',(-0.932386368960449,-0.618937511659511,
58.7773861339448));
#42315=CARTESIAN_POINT('Ctrl Pts',(-0.523540251926434,-0.989107470892482,
58.8011614992419));
#42316=CARTESIAN_POINT('Ctrl Pts',(0.0124596585054514,-1.11904992796231,
58.8249368645392));
#42317=CARTESIAN_POINT('Ctrl Pts',(0.545433454254506,-0.977205368048354,
58.8487122298363));
#42318=CARTESIAN_POINT('Ctrl Pts',(0.945936188801736,-0.598024005436041,
58.8724875951334));
#42319=CARTESIAN_POINT('Ctrl Pts',(1.11669656012879,-0.073598756504813,
58.8962629604306));
#42320=CARTESIAN_POINT('Ctrl Pts',(1.01624148398594,0.468701643466889,58.9200383257278));
#42321=CARTESIAN_POINT('Ctrl Pts',(0.668968786425046,0.897167067580795,
58.9438136910249));
#42322=CARTESIAN_POINT('Ctrl Pts',(0.15922163050928,1.10773483141972,58.9675890563221));
#42323=CARTESIAN_POINT('Ctrl Pts',(-0.389196161018078,1.04926370975618,
58.9913644216192));
#42324=CARTESIAN_POINT('Ctrl Pts',(-0.843088711998524,0.735954759522071,
59.0151397869164));
#42325=CARTESIAN_POINT('Ctrl Pts',(-1.0922177753444,0.243902266459851,59.0389151522135));
#42326=CARTESIAN_POINT('Ctrl Pts',(-1.07607662720109,-0.307387502598993,
59.0626905175107));
#42327=CARTESIAN_POINT('Ctrl Pts',(-0.798585516696848,-0.784021145687122,
59.0864658828079));
#42328=CARTESIAN_POINT('Ctrl Pts',(-0.327139543262851,-1.07023721837558,
59.110241248105));
#42329=CARTESIAN_POINT('Ctrl Pts',(0.223759793581615,-1.09652156346277,
59.1340166134021));
#42330=CARTESIAN_POINT('Ctrl Pts',(0.720313917313741,-0.856490423114379,
59.1577919786993));
#42331=CARTESIAN_POINT('Ctrl Pts',(1.04192323654097,-0.408440881301712,
59.1815673439965));
#42332=CARTESIAN_POINT('Ctrl Pts',(1.11047752997392,0.138807924073182,59.2053427092936));
#42333=CARTESIAN_POINT('Ctrl Pts',(0.909326810469135,0.652344032029584,
59.2291180745908));
#42334=CARTESIAN_POINT('Ctrl Pts',(0.487325157413065,1.00744338566233,59.2528934398879));
#42335=CARTESIAN_POINT('Ctrl Pts',(-0.0530346202668054,1.11786193844124,
59.2766688051851));
#42336=CARTESIAN_POINT('Ctrl Pts',(-0.580513720437941,0.956782004819481,
59.3004441704822));
#42337=CARTESIAN_POINT('Ctrl Pts',(-0.967001709796653,0.563325552066532,
59.3242195357794));
#42338=CARTESIAN_POINT('Ctrl Pts',(-1.11863108958631,0.0330525305790881,
59.3479949010765));
#42339=CARTESIAN_POINT('Ctrl Pts',(-0.99857517691829,-0.505248058281805,
59.3717702663737));
#42340=CARTESIAN_POINT('Ctrl Pts',(-0.635992311906835,-0.920837533752328,
59.3955456316709));
#42341=CARTESIAN_POINT('Ctrl Pts',(-0.118944083910845,-1.11278043174102,
59.419320996968));
#42342=CARTESIAN_POINT('Ctrl Pts',(0.426992450901576,-1.03445900411316,
59.4430963622652));
#42343=CARTESIAN_POINT('Ctrl Pts',(0.869224046902271,-0.704895411260545,
59.4668717275623));
#42344=CARTESIAN_POINT('Ctrl Pts',(1.10034458760252,-0.204131752730095,
59.4906470928595));
#42345=CARTESIAN_POINT('Ctrl Pts',(1.06422113433627,0.3462099975799,59.5144224581566));
#42346=CARTESIAN_POINT('Ctrl Pts',(0.769627096092177,0.812466686178068,
59.5381978234538));
#42347=CARTESIAN_POINT('Ctrl Pts',(0.288111417332764,1.0813971500596,59.5619731887509));
#42348=CARTESIAN_POINT('Ctrl Pts',(-0.263378754924248,1.08768544121352,
59.5857485540481));
#42349=CARTESIAN_POINT('Ctrl Pts',(-0.750901320154641,0.82980430032555,
59.6095239193452));
#42350=CARTESIAN_POINT('Ctrl Pts',(-1.05605026480425,0.370386101406355,
59.6332992846424));
#42351=CARTESIAN_POINT('Ctrl Pts',(-1.10471302727964,-0.178988892410047,
59.6570746499396));
#42352=CARTESIAN_POINT('Ctrl Pts',(-0.885070996868774,-0.684892294832443,
59.6808500152367));
#42353=CARTESIAN_POINT('Ctrl Pts',(-0.450468731436616,-1.02445389535057,
59.7046253805338));
#42354=CARTESIAN_POINT('Ctrl Pts',(0.0935394015687504,-1.11520320243905,
59.728400745831));
#42355=CARTESIAN_POINT('Ctrl Pts',(0.614831124036485,-0.935099979817495,
59.7521761111282));
#42356=CARTESIAN_POINT('Ctrl Pts',(0.986793137377364,-0.527885776223916,
59.7759514764253));
#42357=CARTESIAN_POINT('Ctrl Pts',(1.11909807483697,0.00753651378501131,
59.7997268417225));
#42358=CARTESIAN_POINT('Ctrl Pts',(0.979586733099938,0.541130030933556,
59.8235022070196));
#42359=CARTESIAN_POINT('Ctrl Pts',(0.602199932723299,0.943290627360923,
59.8472775723168));
#42360=CARTESIAN_POINT('Ctrl Pts',(0.07847720070704,1.11635106578832,59.8710529376139));
#42361=CARTESIAN_POINT('Ctrl Pts',(-0.283232877717969,1.05091724415087,
59.8869031811454));
#42362=CARTESIAN_POINT('Ctrl Pts',(-0.44539676218196,0.976988792086596,
59.8948283029111));
#42363=CARTESIAN_POINT('Ctrl Pts',(-0.487177848858668,1.02066752383254,
56.0287216970889));
#42364=CARTESIAN_POINT('Ctrl Pts',(-0.656591676070983,0.939804106528635,
56.0366468188546));
#42365=CARTESIAN_POINT('Ctrl Pts',(-0.954188029735873,0.692125304549036,
56.052497062386));
#42366=CARTESIAN_POINT('Ctrl Pts',(-1.16891903122754,0.152279013351406,
56.0762724276832));
#42367=CARTESIAN_POINT('Ctrl Pts',(-1.09969822348802,-0.424489144743217,
56.1000477929803));
#42368=CARTESIAN_POINT('Ctrl Pts',(-0.763411594228405,-0.898197172052492,
56.1238231582775));
#42369=CARTESIAN_POINT('Ctrl Pts',(-0.241702335063995,-1.15374206193584,
56.1475985235747));
#42370=CARTESIAN_POINT('Ctrl Pts',(0.338705156167176,-1.12908163778266,
56.1713738888718));
#42371=CARTESIAN_POINT('Ctrl Pts',(0.836852543534731,-0.830194377764544,
56.195149254169));
#42372=CARTESIAN_POINT('Ctrl Pts',(1.1317500111436,-0.329676906362474,56.2189246194661));
#42373=CARTESIAN_POINT('Ctrl Pts',(1.1517764336156,0.250910919304856,56.2426999847633));
#42374=CARTESIAN_POINT('Ctrl Pts',(0.892067232420471,0.770558914997795,
56.2664753500605));
#42375=CARTESIAN_POINT('Ctrl Pts',(0.415699086303556,1.10305911090171,56.2902507153576));
#42376=CARTESIAN_POINT('Ctrl Pts',(-0.161631193229248,1.167655954137,56.3140260806548));
#42377=CARTESIAN_POINT('Ctrl Pts',(-0.699705597230648,0.948660722897936,
56.3378014459519));
#42378=CARTESIAN_POINT('Ctrl Pts',(-1.06784041161392,0.499261396849246,
56.3615768112491));
#42379=CARTESIAN_POINT('Ctrl Pts',(-1.17662561327687,-0.0713950368096213,
56.3853521765462));
#42380=CARTESIAN_POINT('Ctrl Pts',(-0.999640220555501,-0.62471154685274,
56.4091275418434));
#42381=CARTESIAN_POINT('Ctrl Pts',(-0.579869204097866,-1.02630248565988,
56.4329029071405));
#42382=CARTESIAN_POINT('Ctrl Pts',(-0.0192636129259017,-1.17863225808771,
56.4566782724377));
#42383=CARTESIAN_POINT('Ctrl Pts',(0.546020589995489,-1.04470407372333,
56.4804536377348));
#42384=CARTESIAN_POINT('Ctrl Pts',(0.978691132191524,-0.657045473443933,
56.5042290030319));
#42385=CARTESIAN_POINT('Ctrl Pts',(1.17366401973703,-0.109808265570952,
56.5280043683291));
#42386=CARTESIAN_POINT('Ctrl Pts',(1.08358560177813,0.464098405527887,56.5517797336263));
#42387=CARTESIAN_POINT('Ctrl Pts',(0.730333494260416,0.925288103008396,
56.5755550989234));
#42388=CARTESIAN_POINT('Ctrl Pts',(0.199703097486968,1.16175029987297,56.5993304642206));
#42389=CARTESIAN_POINT('Ctrl Pts',(-0.379429790363681,1.11605471218396,
56.6231058295178));
#42390=CARTESIAN_POINT('Ctrl Pts',(-0.866409425441811,0.799299564561584,
56.6468811948149));
#42391=CARTESIAN_POINT('Ctrl Pts',(-1.14296160116897,0.288416131060683,
56.6706565601121));
#42392=CARTESIAN_POINT('Ctrl Pts',(-1.14191926002402,-0.292515794426723,
56.6944319254092));
#42393=CARTESIAN_POINT('Ctrl Pts',(-0.863535558531093,-0.802403530373075,
56.7182072907064));
#42394=CARTESIAN_POINT('Ctrl Pts',(-0.375422382375764,-1.11740911094109,
56.7419826560035));
#42395=CARTESIAN_POINT('Ctrl Pts',(0.203870755339166,-1.1610261846833,56.7657580213007));
#42396=CARTESIAN_POINT('Ctrl Pts',(0.733649190394879,-0.92266134189949,
56.7895333865978));
#42397=CARTESIAN_POINT('Ctrl Pts',(1.08524404312101,-0.460206967866842,
56.813308751895));
#42398=CARTESIAN_POINT('Ctrl Pts',(1.17326241564812,0.114019254647519,56.8370841171921));
#42399=CARTESIAN_POINT('Ctrl Pts',(0.976327021484194,0.660553278337659,
56.8608594824893));
#42400=CARTESIAN_POINT('Ctrl Pts',(0.542268151290001,1.04665674339745,56.8846348477864));
#42401=CARTESIAN_POINT('Ctrl Pts',(-0.0234930134682861,1.17855554163603,
56.9084102130836));
#42402=CARTESIAN_POINT('Ctrl Pts',(-0.583548359486088,1.02421501577741,
56.9321855783807));
#42403=CARTESIAN_POINT('Ctrl Pts',(-1.00187556279331,0.62112031288665,56.9559609436779));
#42404=CARTESIAN_POINT('Ctrl Pts',(-1.17687423910946,0.067172254118474,
56.979736308975));
#42405=CARTESIAN_POINT('Ctrl Pts',(-1.06604193432269,-0.503090131754104,
57.0035116742722));
#42406=CARTESIAN_POINT('Ctrl Pts',(-0.69629682317279,-0.951165506335416,
57.0272870395694));
#42407=CARTESIAN_POINT('Ctrl Pts',(-0.157440011305465,-1.1682284576413,
57.0510624048665));
#42408=CARTESIAN_POINT('Ctrl Pts',(0.419654728966468,-1.10156025475636,
57.0748377701637));
#42409=CARTESIAN_POINT('Ctrl Pts',(0.894826664813918,-0.767352804348056,
57.0986131354608));
#42410=CARTESIAN_POINT('Ctrl Pts',(1.1526693610356,-0.246776073663168,57.122388500758));
#42411=CARTESIAN_POINT('Ctrl Pts',(1.13055978758964,0.333735903205072,57.1461638660551));
#42412=CARTESIAN_POINT('Ctrl Pts',(0.833867762983234,0.833192438912023,
57.1699392313523));
#42413=CARTESIAN_POINT('Ctrl Pts',(0.334651770324009,1.13028902455161,57.1937145966494));
#42414=CARTESIAN_POINT('Ctrl Pts',(-0.245842102894417,1.15286892006302,
57.2174899619466));
#42415=CARTESIAN_POINT('Ctrl Pts',(-0.766627566215206,0.895448078406435,
57.2412653272437));
#42416=CARTESIAN_POINT('Ctrl Pts',(-1.10121989002294,0.420547072538497,
57.2650406925409));
#42417=CARTESIAN_POINT('Ctrl Pts',(-1.16835563171236,-0.156493463917345,
57.288816057838));
#42418=CARTESIAN_POINT('Ctrl Pts',(-0.951729332062369,-0.695525962775614,
57.3125914231352));
#42419=CARTESIAN_POINT('Ctrl Pts',(-0.50395367108924,-1.06563398209634,
57.3363667884324));
#42420=CARTESIAN_POINT('Ctrl Pts',(0.0662187315670568,-1.1769282756364,
57.3601421537296));
#42421=CARTESIAN_POINT('Ctrl Pts',(0.620308392004842,-1.00237846405995,
57.3839175190267));
#42422=CARTESIAN_POINT('Ctrl Pts',(1.02374189022832,-0.584377984351374,
57.4076928843239));
#42423=CARTESIAN_POINT('Ctrl Pts',(1.17853612084276,-0.0244478684494714,
57.431468249621));
#42424=CARTESIAN_POINT('Ctrl Pts',(1.04709574414639,0.541419974690026,57.4552436149181));
#42425=CARTESIAN_POINT('Ctrl Pts',(0.661344079198414,0.975791522463701,
57.4790189802153));
#42426=CARTESIAN_POINT('Ctrl Pts',(0.114969791439926,1.17316965246254,57.5027943455124));
#42427=CARTESIAN_POINT('Ctrl Pts',(-0.459327554868421,1.08561654544384,
57.5265697108096));
#42428=CARTESIAN_POINT('Ctrl Pts',(-0.922066638371227,0.734396487468189,
57.5503450761068));
#42429=CARTESIAN_POINT('Ctrl Pts',(-1.16086062805725,0.204811348878305,
57.5741204414039));
#42430=CARTESIAN_POINT('Ctrl Pts',(-1.11771291045225,-0.374516937148636,
57.5978958067011));
#42431=CARTESIAN_POINT('Ctrl Pts',(-0.80310290132176,-0.862885169817746,
57.6216711719983));
#42432=CARTESIAN_POINT('Ctrl Pts',(-0.293440878490046,-1.14168188968461,
57.6454465372954));
#42433=CARTESIAN_POINT('Ctrl Pts',(0.28749001182744,-1.14319490005085,57.6692219025925));
#42434=CARTESIAN_POINT('Ctrl Pts',(0.798597339518466,-0.867056731544629,
57.6929972678897));
#42435=CARTESIAN_POINT('Ctrl Pts',(1.11574693283554,-0.380333890510585,
57.7167726331868));
#42436=CARTESIAN_POINT('Ctrl Pts',(1.16191171751556,0.198761784815075,57.740547998484));
#42437=CARTESIAN_POINT('Ctrl Pts',(0.925879513650944,0.72958358849711,57.7643233637812));
#42438=CARTESIAN_POINT('Ctrl Pts',(0.464976171498692,1.08320923479319,57.7880987290783));
#42439=CARTESIAN_POINT('Ctrl Pts',(-0.108857329945276,1.17375260090021,
57.8118740943755));
#42440=CARTESIAN_POINT('Ctrl Pts',(-0.656252324720897,0.979223147551796,
57.8356494596726));
#42441=CARTESIAN_POINT('Ctrl Pts',(-1.04426134638865,0.54686682733678,57.8594248249698));
#42442=CARTESIAN_POINT('Ctrl Pts',(-1.17864747850111,-0.0183086817055737,
57.8832001902669));
#42443=CARTESIAN_POINT('Ctrl Pts',(-1.02677195753382,-0.579037506233389,
57.9069755555641));
#42444=CARTESIAN_POINT('Ctrl Pts',(-0.625521247410444,-0.999133752528114,
57.9307509208612));
#42445=CARTESIAN_POINT('Ctrl Pts',(-0.0723483132239842,-1.17656738352568,
57.9545262861584));
#42446=CARTESIAN_POINT('Ctrl Pts',(0.498396073087726,-1.06824456035758,
57.9783016514556));
#42447=CARTESIAN_POINT('Ctrl Pts',(0.948093508234708,-0.700473972425836,
58.0020770167527));
#42448=CARTESIAN_POINT('Ctrl Pts',(1.16752462551148,-0.162577166991841,
58.0258523820499));
#42449=CARTESIAN_POINT('Ctrl Pts',(1.10339553042073,0.414805243277359,58.049627747347));
#42450=CARTESIAN_POINT('Ctrl Pts',(0.771281448893881,0.89144265827645,58.0734031126442));
#42451=CARTESIAN_POINT('Ctrl Pts',(0.251843925390228,1.15157271748113,58.0971784779413));
#42452=CARTESIAN_POINT('Ctrl Pts',(-0.328759688666628,1.13201685213191,
58.1209538432385));
#42453=CARTESIAN_POINT('Ctrl Pts',(-0.829516449732817,0.837524653980699,
58.1447292085356));
#42454=CARTESIAN_POINT('Ctrl Pts',(-1.12880605926414,0.339620327676922,
58.1685045738328));
#42455=CARTESIAN_POINT('Ctrl Pts',(-1.15393915090063,-0.240768607633033,
58.1922799391299));
#42456=CARTESIAN_POINT('Ctrl Pts',(-0.898811575191243,-0.762681348077337,
58.2160553044271));
#42457=CARTESIAN_POINT('Ctrl Pts',(-0.42538693270437,-1.09935937885989,
58.2398306697243));
#42458=CARTESIAN_POINT('Ctrl Pts',(0.151352711745039,-1.16903269545819,
58.2636060350214));
#42459=CARTESIAN_POINT('Ctrl Pts',(0.691332868516809,-0.954779530211634,
58.2873814003186));
#42460=CARTESIAN_POINT('Ctrl Pts',(1.06340693514731,-0.508636192856387,
58.3111567656157));
#42461=CARTESIAN_POINT('Ctrl Pts',(1.17720816557841,0.0610411443072006,
58.3349321309129));
#42462=CARTESIAN_POINT('Ctrl Pts',(1.00509731318217,0.615893235420565,58.35870749621));
#42463=CARTESIAN_POINT('Ctrl Pts',(0.588875457601626,1.02116148665983,58.3824828615072));
#42464=CARTESIAN_POINT('Ctrl Pts',(0.029631650991658,1.17841718065477,58.4062582268043));
#42465=CARTESIAN_POINT('Ctrl Pts',(-0.536808883691014,1.04946715469958,
58.4300335921015));
#42466=CARTESIAN_POINT('Ctrl Pts',(-0.972873032527844,0.66562988888939,
58.4538089573986));
#42467=CARTESIAN_POINT('Ctrl Pts',(-1.17265258600602,0.120129092796946,
58.4775843226958));
#42468=CARTESIAN_POINT('Ctrl Pts',(-1.08762648394992,-0.4545478168615,58.5013596879929));
#42469=CARTESIAN_POINT('Ctrl Pts',(-0.738445271135204,-0.918827333039719,
58.5251350532901));
#42470=CARTESIAN_POINT('Ctrl Pts',(-0.20991563745684,-1.15994849521602,
58.5489104185873));
#42471=CARTESIAN_POINT('Ctrl Pts',(0.369596837555985,-1.11934948254397,
58.5726857838844));
#42472=CARTESIAN_POINT('Ctrl Pts',(0.859344218576179,-0.806890699167193,
58.5964611491816));
#42473=CARTESIAN_POINT('Ctrl Pts',(1.14038008825714,-0.298459948250121,
58.6202365144787));
#42474=CARTESIAN_POINT('Ctrl Pts',(1.14444842086004,0.282458666699742,58.6440118797758));
#42475=CARTESIAN_POINT('Ctrl Pts',(0.870561128226679,0.794775696925566,
58.6677872450731));
#42476=CARTESIAN_POINT('Ctrl Pts',(0.385238039718154,1.11406316659198,58.6915626103702));
#42477=CARTESIAN_POINT('Ctrl Pts',(-0.193648968529259,1.16277476898597,
58.7153379756674));
#42478=CARTESIAN_POINT('Ctrl Pts',(-0.72550387018033,0.929079770932609,
58.7391133409644));
#42479=CARTESIAN_POINT('Ctrl Pts',(-1.08115346788616,0.469736378493884,
58.7628887062617));
#42480=CARTESIAN_POINT('Ctrl Pts',(-1.17422007568598,-0.103693299006395,
58.7866640715588));
#42481=CARTESIAN_POINT('Ctrl Pts',(-0.98210032702512,-0.651938673542211,
58.810439436856));
#42482=CARTESIAN_POINT('Ctrl Pts',(-0.551454922277587,-1.04184574438764,
58.8342148021531));
#42483=CARTESIAN_POINT('Ctrl Pts',(0.0131239956955444,-1.17871661019085,
58.8579901674503));
#42484=CARTESIAN_POINT('Ctrl Pts',(0.574515449417203,-1.02930903269318,
58.8817655327474));
#42485=CARTESIAN_POINT('Ctrl Pts',(0.996372610426357,-0.629910078975558,
58.9055408980446));
#42486=CARTESIAN_POINT('Ctrl Pts',(1.17623776301348,-0.0775229724911266,
58.9293162633417));
#42487=CARTESIAN_POINT('Ctrl Pts',(1.07042651735873,0.493692371156451,58.9530916286389));
#42488=CARTESIAN_POINT('Ctrl Pts',(0.704637568490134,0.945003165854559,
58.976866993936));
#42489=CARTESIAN_POINT('Ctrl Pts',(0.167711177038103,1.16679820341794,59.0006423592332));
#42490=CARTESIAN_POINT('Ctrl Pts',(-0.40994773168867,1.10520945692938,59.0244177245303));
#42491=CARTESIAN_POINT('Ctrl Pts',(-0.888041403574033,0.775195170225595,
59.0481930898275));
#42492=CARTESIAN_POINT('Ctrl Pts',(-1.15045379260996,0.25690690429061,59.0719684551246));
#42493=CARTESIAN_POINT('Ctrl Pts',(-1.13345201373606,-0.323777113089378,
59.0957438204218));
#42494=CARTESIAN_POINT('Ctrl Pts',(-0.841165340050963,-0.825824410573927,
59.119519185719));
#42495=CARTESIAN_POINT('Ctrl Pts',(-0.344582313852902,-1.12730125316288,
59.1432945510161));
#42496=CARTESIAN_POINT('Ctrl Pts',(0.235690453836842,-1.15498705463438,
59.1670699163133));
#42497=CARTESIAN_POINT('Ctrl Pts',(0.758720373125246,-0.902157681232892,
59.1908452816104));
#42498=CARTESIAN_POINT('Ctrl Pts',(1.09747759663501,-0.430218562229815,
59.2146206469076));
#42499=CARTESIAN_POINT('Ctrl Pts',(1.16968714006124,0.146209031110073,59.2383960122047));
#42500=CARTESIAN_POINT('Ctrl Pts',(0.957811254716368,0.687126397936767,
59.2621713775019));
#42501=CARTESIAN_POINT('Ctrl Pts',(0.513308873226614,1.0611593127658,59.285946742799));
#42502=CARTESIAN_POINT('Ctrl Pts',(-0.0558623759866322,1.17746527819375,
59.3097221080962));
#42503=CARTESIAN_POINT('Ctrl Pts',(-0.611466162166566,1.00779671508134,
59.3334974733933));
#42504=CARTESIAN_POINT('Ctrl Pts',(-1.0185613250481,0.593361536937717,59.3572728386905));
#42505=CARTESIAN_POINT('Ctrl Pts',(-1.17827543974936,0.0348148602032075,
59.3810482039876));
#42506=CARTESIAN_POINT('Ctrl Pts',(-1.05181825953123,-0.532187406193635,
59.4048235692848));
#42507=CARTESIAN_POINT('Ctrl Pts',(-0.669902819584936,-0.969935718862406,
59.428598934582));
#42508=CARTESIAN_POINT('Ctrl Pts',(-0.125286069804721,-1.17211283036932,
59.4523742998791));
#42509=CARTESIAN_POINT('Ctrl Pts',(0.449759283949248,-1.08961537840405,
59.4761496651763));
#42510=CARTESIAN_POINT('Ctrl Pts',(0.915570249780245,-0.742479766933245,
59.4999250304734));
#42511=CARTESIAN_POINT('Ctrl Pts',(1.15901391880021,-0.215015864438216,
59.5237003957705));
#42512=CARTESIAN_POINT('Ctrl Pts',(1.12096439722085,0.364669586731168,59.5474757610677));
#42513=CARTESIAN_POINT('Ctrl Pts',(0.810662883888195,0.855786640341092,
59.5712511263649));
#42514=CARTESIAN_POINT('Ctrl Pts',(0.303473245214488,1.13905622183395,59.5950264916621));
#42515=CARTESIAN_POINT('Ctrl Pts',(-0.277421860672377,1.14567979871612,
59.6188018569592));
#42516=CARTESIAN_POINT('Ctrl Pts',(-0.790938667314156,0.874048679653256,
59.6425772222563));
#42517=CARTESIAN_POINT('Ctrl Pts',(-1.11235786466458,0.39013473751478,59.6663525875535));
#42518=CARTESIAN_POINT('Ctrl Pts',(-1.16361527954326,-0.188532410620455,
59.6901279528507));
#42519=CARTESIAN_POINT('Ctrl Pts',(-0.932262144109214,-0.721410103283539,
59.7139033181478));
#42520=CARTESIAN_POINT('Ctrl Pts',(-0.474487297526397,-1.07907680671876,
59.737678683445));
#42521=CARTESIAN_POINT('Ctrl Pts',(0.0985268338626855,-1.1746647809062,
59.7614540487421));
#42522=CARTESIAN_POINT('Ctrl Pts',(0.647613337220575,-0.984958625042814,
59.7852294140393));
#42523=CARTESIAN_POINT('Ctrl Pts',(1.03940801280157,-0.556032145814661,
59.8090047793364));
#42524=CARTESIAN_POINT('Ctrl Pts',(1.17876732421126,0.00793835356166478,
59.8327801446336));
#42525=CARTESIAN_POINT('Ctrl Pts',(1.03181736987376,0.569982571640854,59.8565555099308));
#42526=CARTESIAN_POINT('Ctrl Pts',(0.634308662750459,0.993585990155316,
59.8803308752279));
#42527=CARTESIAN_POINT('Ctrl Pts',(0.0826615307175012,1.17587384724203,
59.9041062405251));
#42528=CARTESIAN_POINT('Ctrl Pts',(-0.298334586488231,1.10695115621182,
59.9199564840565));
#42529=CARTESIAN_POINT('Ctrl Pts',(-0.469144895675092,1.02908090910628,
59.9278816058222));
#42530=CARTESIAN_POINT('Ctrl Pts',(-0.511838811167433,1.07233375495119,
56.061775));
#42531=CARTESIAN_POINT('Ctrl Pts',(-0.689828373128885,0.987377028210164,
56.0697001217657));
#42532=CARTESIAN_POINT('Ctrl Pts',(-1.00248906618882,0.727160715310048,
56.0855503652972));
#42533=CARTESIAN_POINT('Ctrl Pts',(-1.22808975961479,0.159987383133561,
56.1093257305943));
#42534=CARTESIAN_POINT('Ctrl Pts',(-1.15536499180269,-0.445976802327642,
56.1331010958914));
#42535=CARTESIAN_POINT('Ctrl Pts',(-0.802055519840889,-0.943663949036954,
56.1568764611886));
#42536=CARTESIAN_POINT('Ctrl Pts',(-0.25393731698881,-1.21214453152697,
56.1806518264858));
#42537=CARTESIAN_POINT('Ctrl Pts',(0.355850424798725,-1.18623579571104,
56.2044271917829));
#42538=CARTESIAN_POINT('Ctrl Pts',(0.879214052955683,-0.87221885056635,
56.2282025570801));
#42539=CARTESIAN_POINT('Ctrl Pts',(1.18903924223887,-0.346365164625703,
56.2519779223772));
#42540=CARTESIAN_POINT('Ctrl Pts',(1.21007940302208,0.263612040134405,56.2757532876744));
#42541=CARTESIAN_POINT('Ctrl Pts',(0.937223711614153,0.809564638275162,
56.2995286529715));
#42542=CARTESIAN_POINT('Ctrl Pts',(0.436741790776142,1.15889600747247,56.3233040182687));
#42543=CARTESIAN_POINT('Ctrl Pts',(-0.169812970733057,1.22676274551112,
56.3470793835658));
#42544=CARTESIAN_POINT('Ctrl Pts',(-0.735124722712158,0.996681966856387,
56.370854748863));
#42545=CARTESIAN_POINT('Ctrl Pts',(-1.12189453620986,0.524534028843431,
56.3946301141602));
#42546=CARTESIAN_POINT('Ctrl Pts',(-1.23618644915751,-0.0750090564451986,
56.4184054794573));
#42547=CARTESIAN_POINT('Ctrl Pts',(-1.05024204873632,-0.656334470487052,
56.4421808447545));
#42548=CARTESIAN_POINT('Ctrl Pts',(-0.60922220653789,-1.07825395877292,
56.4659562100516));
#42549=CARTESIAN_POINT('Ctrl Pts',(-0.0202387377872045,-1.2382946704094,
56.4897315753488));
#42550=CARTESIAN_POINT('Ctrl Pts',(0.573660174227889,-1.09758703596446,
56.513506940646));
#42551=CARTESIAN_POINT('Ctrl Pts',(1.02823251667656,-0.690305141743117,
56.5372823059431));
#42552=CARTESIAN_POINT('Ctrl Pts',(1.23307493963353,-0.115366764391829,
56.5610576712402));
#42553=CARTESIAN_POINT('Ctrl Pts',(1.13843674853363,0.487591085486743,56.5848330365374));
#42554=CARTESIAN_POINT('Ctrl Pts',(0.767303005121764,0.972126224007736,
56.6086084018345));
#42555=CARTESIAN_POINT('Ctrl Pts',(0.209812076315972,1.22055814679065,56.6323837671317));
#42556=CARTESIAN_POINT('Ctrl Pts',(-0.398636541616641,1.17254944661446,
56.6561591324289));
#42557=CARTESIAN_POINT('Ctrl Pts',(-0.910267105413995,0.839760140676135,
56.679934497726));
#42558=CARTESIAN_POINT('Ctrl Pts',(-1.20081836340238,0.303015767218183,
56.7037098630232));
#42559=CARTESIAN_POINT('Ctrl Pts',(-1.19972325890673,-0.307322955708736,
56.7274852283203));
#42560=CARTESIAN_POINT('Ctrl Pts',(-0.907247763244644,-0.843021229361873,
56.7512605936174));
#42561=CARTESIAN_POINT('Ctrl Pts',(-0.394426278475162,-1.17397240509116,
56.7750359589146));
#42562=CARTESIAN_POINT('Ctrl Pts',(0.21419070117631,-1.21979737686095,56.7988113242118));
#42563=CARTESIAN_POINT('Ctrl Pts',(0.770786541927939,-0.969366496145824,
56.8225866895089));
#42564=CARTESIAN_POINT('Ctrl Pts',(1.140179140244,-0.483502663094748,56.8463620548061));
#42565=CARTESIAN_POINT('Ctrl Pts',(1.23265300632948,0.119790913904855,56.8701374201032));
#42566=CARTESIAN_POINT('Ctrl Pts',(1.02574873459012,0.693990511861678,56.8939127854004));
#42567=CARTESIAN_POINT('Ctrl Pts',(0.569717786924172,1.09963854985604,56.9176881506976));
#42568=CARTESIAN_POINT('Ctrl Pts',(-0.0246822307551888,1.23821407056785,
56.9414635159947));
#42569=CARTESIAN_POINT('Ctrl Pts',(-0.613087600919873,1.07606082108103,
56.9652388812919));
#42570=CARTESIAN_POINT('Ctrl Pts',(-1.05259054408814,0.652561448113126,
56.989014246589));
#42571=CARTESIAN_POINT('Ctrl Pts',(-1.23644766043974,0.0705725163243472,
57.0127896118862));
#42572=CARTESIAN_POINT('Ctrl Pts',(-1.1200050199258,-0.528556574463199,
57.0365649771833));
#42573=CARTESIAN_POINT('Ctrl Pts',(-0.73154339637436,-0.999313542532237,
57.0603403424805));
#42574=CARTESIAN_POINT('Ctrl Pts',(-0.165409631011685,-1.22736422916583,
57.0841157077776));
#42575=CARTESIAN_POINT('Ctrl Pts',(0.440897668229782,-1.15732127916876,
57.1078910730748));
#42576=CARTESIAN_POINT('Ctrl Pts',(0.940122826586366,-0.806196234175355,
57.1316664383719));
#42577=CARTESIAN_POINT('Ctrl Pts',(1.211017530464,-0.259267888439993,57.1554418036691));
#42578=CARTESIAN_POINT('Ctrl Pts',(1.18778876952072,0.350629628051763,57.1792171689663));
#42579=CARTESIAN_POINT('Ctrl Pts',(0.876078182692593,0.875368673689724,
57.2029925342634));
#42580=CARTESIAN_POINT('Ctrl Pts',(0.351591856401113,1.18750430044682,57.2267678995605));
#42581=CARTESIAN_POINT('Ctrl Pts',(-0.258286640033346,1.21122719117742,
57.2505432648577));
#42582=CARTESIAN_POINT('Ctrl Pts',(-0.805434284459037,0.940775696159941,
57.2743186301548));
#42583=CARTESIAN_POINT('Ctrl Pts',(-1.15696368515882,0.441835182269334,
57.298093995452));
#42584=CARTESIAN_POINT('Ctrl Pts',(-1.22749784079349,-0.16441516935669,
57.3218693607492));
#42585=CARTESIAN_POINT('Ctrl Pts',(-0.999905909140176,-0.73073351499286,
57.3456447260463));
#42586=CARTESIAN_POINT('Ctrl Pts',(-0.529463826194227,-1.11957641714134,
57.3694200913435));
#42587=CARTESIAN_POINT('Ctrl Pts',(0.0695707264230086,-1.23650443229785,
57.3931954566407));
#42588=CARTESIAN_POINT('Ctrl Pts',(0.651708427763611,-1.05311890223713,
57.4169708219377));
#42589=CARTESIAN_POINT('Ctrl Pts',(1.0755637458976,-0.613959221429223,57.440746187235));
#42590=CARTESIAN_POINT('Ctrl Pts',(1.23819366669324,-0.0256854205339441,
57.4645215525321));
#42591=CARTESIAN_POINT('Ctrl Pts',(1.10009977284055,0.568826675590577,57.4882969178293));
#42592=CARTESIAN_POINT('Ctrl Pts',(0.694821343093825,1.02518612858766,57.5120722831264));
#42593=CARTESIAN_POINT('Ctrl Pts',(0.120789566907943,1.23255554746772,57.5358476484236));
#42594=CARTESIAN_POINT('Ctrl Pts',(-0.482578734174961,1.14057049864941,
57.5596230137207));
#42595=CARTESIAN_POINT('Ctrl Pts',(-0.96874168870103,0.771571667209171,
57.5833983790179));
#42596=CARTESIAN_POINT('Ctrl Pts',(-1.21962343975183,0.215178907598248,
57.607173744315));
#42597=CARTESIAN_POINT('Ctrl Pts',(-1.1742915829458,-0.393474999574203,
57.6309491096122));
#42598=CARTESIAN_POINT('Ctrl Pts',(-0.843756002496121,-0.906564451828457,
57.6547244749094));
#42599=CARTESIAN_POINT('Ctrl Pts',(-0.308294867564569,-1.19947387287119,
57.6784998402065));
#42600=CARTESIAN_POINT('Ctrl Pts',(0.302042767792087,-1.20106347188305,
57.7022752055036));
#42601=CARTESIAN_POINT('Ctrl Pts',(0.839022368973077,-0.910947178177785,
57.7260505708008));
#42602=CARTESIAN_POINT('Ctrl Pts',(1.17222608746303,-0.399586407349361,
57.7498259360979));
#42603=CARTESIAN_POINT('Ctrl Pts',(1.2207277354008,0.208823114358751,57.7736013013951));
#42604=CARTESIAN_POINT('Ctrl Pts',(0.972747571880807,0.766515139098543,
57.7973766666923));
#42605=CARTESIAN_POINT('Ctrl Pts',(0.488513284006311,1.13804132983677,57.8211520319894));
#42606=CARTESIAN_POINT('Ctrl Pts',(-0.114367692366517,1.23316800477876,
57.8449273972866));
#42607=CARTESIAN_POINT('Ctrl Pts',(-0.689471843799805,1.02879146267578,
57.8687027625837));
#42608=CARTESIAN_POINT('Ctrl Pts',(-1.09712189775428,0.574549248137447,
57.8924781278809));
#42609=CARTESIAN_POINT('Ctrl Pts',(-1.23831066128074,-0.0192354679100782,
57.916253493178));
#42610=CARTESIAN_POINT('Ctrl Pts',(-1.07874719533202,-0.608348408094048,
57.9400288584752));
#42611=CARTESIAN_POINT('Ctrl Pts',(-0.657185158119568,-1.04970994327701,
57.9638042237723));
#42612=CARTESIAN_POINT('Ctrl Pts',(-0.0760105877500149,-1.23612527181397,
57.9875795890695));
#42613=CARTESIAN_POINT('Ctrl Pts',(0.523624902358283,-1.12231914297919,
58.0113549543667));
#42614=CARTESIAN_POINT('Ctrl Pts',(0.996086039764082,-0.735931993090646,
58.0351303196638));
#42615=CARTESIAN_POINT('Ctrl Pts',(1.22662476902529,-0.170806829725578,
58.058905684961));
#42616=CARTESIAN_POINT('Ctrl Pts',(1.15924945656108,0.435802701379992,58.0826810502581));
#42617=CARTESIAN_POINT('Ctrl Pts',(0.810323746866142,0.936567521501829,
58.1064564155553));
#42618=CARTESIAN_POINT('Ctrl Pts',(0.26459227502536,1.20986537476868,58.1302317808524));
#42619=CARTESIAN_POINT('Ctrl Pts',(-0.345401517333186,1.18931959072875,
58.1540071461496));
#42620=CARTESIAN_POINT('Ctrl Pts',(-0.871506605790379,0.87992018565947,
58.1777825114468));
#42621=CARTESIAN_POINT('Ctrl Pts',(-1.18594626739684,0.35681192232712,58.2015578767439));
#42622=CARTESIAN_POINT('Ctrl Pts',(-1.21235159714309,-0.252956324237721,
58.2253332420411));
#42623=CARTESIAN_POINT('Ctrl Pts',(-0.944309453287311,-0.80128830860027,
58.2491086073382));
#42624=CARTESIAN_POINT('Ctrl Pts',(-0.446920036351515,-1.15500899484585,
58.2728839726354));
#42625=CARTESIAN_POINT('Ctrl Pts',(0.159014192102606,-1.22820917753338,
58.2966593379325));
#42626=CARTESIAN_POINT('Ctrl Pts',(0.726328166133983,-1.00311050844247,
58.3204347032297));
#42627=CARTESIAN_POINT('Ctrl Pts',(1.11723663698614,-0.534383377401609,
58.3442100685268));
#42628=CARTESIAN_POINT('Ctrl Pts',(1.23679849027999,0.0641310494877601,
58.367985433824));
#42629=CARTESIAN_POINT('Ctrl Pts',(1.0559753796113,0.647069775775413,58.3917607991211));
#42630=CARTESIAN_POINT('Ctrl Pts',(0.618684356956339,1.07285272219666,58.4155361644183));
#42631=CARTESIAN_POINT('Ctrl Pts',(0.0311316063569641,1.23806870574815,
58.4393115297154));
#42632=CARTESIAN_POINT('Ctrl Pts',(-0.563982170979687,1.10259122429135,
58.4630868950126));
#42633=CARTESIAN_POINT('Ctrl Pts',(-1.02211990457384,0.69932410064378,58.4868622603097));
#42634=CARTESIAN_POINT('Ctrl Pts',(-1.23201230708637,0.126210032307217,
58.5106376256069));
#42635=CARTESIAN_POINT('Ctrl Pts',(-1.14268218032353,-0.477557045637837,
58.534412990904));
#42636=CARTESIAN_POINT('Ctrl Pts',(-0.775825400468297,-0.965338409603322,
58.5581883562012));
#42637=CARTESIAN_POINT('Ctrl Pts',(-0.220541575469977,-1.21866513470948,
58.5819637214983));
#42638=CARTESIAN_POINT('Ctrl Pts',(0.388305844342232,-1.17601099838264,
58.6057390867956));
#42639=CARTESIAN_POINT('Ctrl Pts',(0.902844257492586,-0.847735538820877,
58.6295144520926));
#42640=CARTESIAN_POINT('Ctrl Pts',(1.19810617420309,-0.313568002837821,
58.6532898173898));
#42641=CARTESIAN_POINT('Ctrl Pts',(1.20238044596602,0.29675673577161,58.677065182687));
#42642=CARTESIAN_POINT('Ctrl Pts',(0.914628967560865,0.835007274678378,
58.7008405479842));
#42643=CARTESIAN_POINT('Ctrl Pts',(0.404738804787115,1.17045708890448,58.7246159132813));
#42644=CARTESIAN_POINT('Ctrl Pts',(-0.203451487106854,1.22163447457137,
58.7483912785784));
#42645=CARTESIAN_POINT('Ctrl Pts',(-0.762228905276438,0.976109826314818,
58.7721666438755));
#42646=CARTESIAN_POINT('Ctrl Pts',(-1.1358814999262,0.493514452871106,58.7959420091728));
#42647=CARTESIAN_POINT('Ctrl Pts',(-1.23365914315699,-0.108942257973756,
58.8197173744699));
#42648=CARTESIAN_POINT('Ctrl Pts',(-1.03181428508979,-0.684939835424913,
58.8434927397671));
#42649=CARTESIAN_POINT('Ctrl Pts',(-0.57936959262874,-1.09458401788281,
58.8672681050642));
#42650=CARTESIAN_POINT('Ctrl Pts',(0.0137883328856377,-1.23838329241939,
58.8910434703614));
#42651=CARTESIAN_POINT('Ctrl Pts',(0.6035974445799,-1.08141269733801,58.9148188356585));
#42652=CARTESIAN_POINT('Ctrl Pts',(1.04680903205098,-0.661796152515074,
58.9385942009557));
#42653=CARTESIAN_POINT('Ctrl Pts',(1.23577896589818,-0.0814471884774405,
58.9623695662528));
#42654=CARTESIAN_POINT('Ctrl Pts',(1.12461155073152,0.518683098846014,58.98614493155));
#42655=CARTESIAN_POINT('Ctrl Pts',(0.740306350555223,0.992839264128324,
59.0099202968471));
#42656=CARTESIAN_POINT('Ctrl Pts',(0.176200723566927,1.22586157541615,59.0336956621443));
#42657=CARTESIAN_POINT('Ctrl Pts',(-0.430699302359262,1.16115520410258,
59.0574710274414));
#42658=CARTESIAN_POINT('Ctrl Pts',(-0.932994095149541,0.81443558092912,
59.0812463927386));
#42659=CARTESIAN_POINT('Ctrl Pts',(-1.20868980987552,0.269911542121367,
59.1050217580358));
#42660=CARTESIAN_POINT('Ctrl Pts',(-1.19082740027104,-0.340166723579763,
59.1287971233329));
#42661=CARTESIAN_POINT('Ctrl Pts',(-0.883745163405079,-0.867627675460732,
59.1525724886301));
#42662=CARTESIAN_POINT('Ctrl Pts',(-0.362025084442952,-1.18436528795019,
59.1763478539272));
#42663=CARTESIAN_POINT('Ctrl Pts',(0.247621114092068,-1.213452545806,59.2001232192244));
#42664=CARTESIAN_POINT('Ctrl Pts',(0.797126828936751,-0.947824939351406,
59.2238985845215));
#42665=CARTESIAN_POINT('Ctrl Pts',(1.15303195672905,-0.451996243157917,
59.2476739498187));
#42666=CARTESIAN_POINT('Ctrl Pts',(1.22889675014856,0.153610138146963,59.2714493151158));
#42667=CARTESIAN_POINT('Ctrl Pts',(1.0062956989636,0.721908763843951,59.295224680413));
#42668=CARTESIAN_POINT('Ctrl Pts',(0.539292589040162,1.11487523986926,59.3190000457101));
#42669=CARTESIAN_POINT('Ctrl Pts',(-0.0586901317064581,1.23706861794625,
59.3427754110073));
#42670=CARTESIAN_POINT('Ctrl Pts',(-0.642418603895192,1.0588114253432,59.3665507763045));
#42671=CARTESIAN_POINT('Ctrl Pts',(-1.07012094029954,0.623397521808901,
59.3903261416016));
#42672=CARTESIAN_POINT('Ctrl Pts',(-1.2379197899124,0.0365771898273263,
59.4141015068987));
#42673=CARTESIAN_POINT('Ctrl Pts',(-1.10506134214416,-0.559126754105465,
59.4378768721959));
#42674=CARTESIAN_POINT('Ctrl Pts',(-0.703813327263037,-1.01903390397248,
59.4616522374931));
#42675=CARTESIAN_POINT('Ctrl Pts',(-0.131628055698595,-1.23144522899762,
59.4854276027902));
#42676=CARTESIAN_POINT('Ctrl Pts',(0.47252611699692,-1.14477175269494,59.5092029680874));
#42677=CARTESIAN_POINT('Ctrl Pts',(0.961916452658219,-0.780064122605945,
59.5329783333845));
#42678=CARTESIAN_POINT('Ctrl Pts',(1.2176832499979,-0.225899976146337,59.5567536986817));
#42679=CARTESIAN_POINT('Ctrl Pts',(1.17770766010544,0.383129175882436,59.5805290639788));
#42680=CARTESIAN_POINT('Ctrl Pts',(0.851698671684214,0.899106594504114,
59.604304429276));
#42681=CARTESIAN_POINT('Ctrl Pts',(0.318835073096213,1.1967152936083,59.6280797945732));
#42682=CARTESIAN_POINT('Ctrl Pts',(-0.291464966420505,1.20367415621872,
59.6518551598703));
#42683=CARTESIAN_POINT('Ctrl Pts',(-0.830976014473671,0.918293058980961,
59.6756305251674));
#42684=CARTESIAN_POINT('Ctrl Pts',(-1.16866546452492,0.409883373623204,
59.6994058904646));
#42685=CARTESIAN_POINT('Ctrl Pts',(-1.22251753180688,-0.198075928830864,
59.7231812557618));
#42686=CARTESIAN_POINT('Ctrl Pts',(-0.979453291349652,-0.757927911734636,
59.7469566210589));
#42687=CARTESIAN_POINT('Ctrl Pts',(-0.498505863616178,-1.13369971808696,
59.770731986356));
#42688=CARTESIAN_POINT('Ctrl Pts',(0.103514266156622,-1.23412635937334,
59.7945073516532));
#42689=CARTESIAN_POINT('Ctrl Pts',(0.680395550404662,-1.03481727026813,
59.8182827169504));
#42690=CARTESIAN_POINT('Ctrl Pts',(1.09202288822577,-0.584178515405407,
59.8420580822475));
#42691=CARTESIAN_POINT('Ctrl Pts',(1.23843657358556,0.00834019333831885,
59.8658334475447));
#42692=CARTESIAN_POINT('Ctrl Pts',(1.08404800664758,0.598835112348151,59.8896088128419));
#42693=CARTESIAN_POINT('Ctrl Pts',(0.666417392777619,1.04388135294971,59.913384178139));
#42694=CARTESIAN_POINT('Ctrl Pts',(0.0868458607279623,1.23539662869573,
59.9371595434362));
#42695=CARTESIAN_POINT('Ctrl Pts',(-0.313436295258493,1.16298506827277,
59.9530097869676));
#42696=CARTESIAN_POINT('Ctrl Pts',(-0.492893029168225,1.08117302612596,
59.9609349087333));
#42697=CARTESIAN_POINT('Ctrl Pts',(-1.1881744462934,-2.6792430042513E-5,
59.7155118763048));
#42698=CARTESIAN_POINT('Ctrl Pts',(-1.18822732035292,-0.0636541554091953,
59.7180683361238));
#42699=CARTESIAN_POINT('Ctrl Pts',(-1.18320405435424,-0.127273252397746,
59.7206247959428));
#42700=CARTESIAN_POINT('Ctrl Pts',(-1.17303148051702,-0.190058042239148,
59.7231812557618));
#42701=CARTESIAN_POINT('Ctrl Pts',(-1.14149611832114,-0.384693256465457,
59.7311063775275));
#42702=CARTESIAN_POINT('Ctrl Pts',(-1.06047470483539,-0.571310584100047,
59.7390314992932));
#42703=CARTESIAN_POINT('Ctrl Pts',(-0.939806093470275,-0.727247882309399,
59.7469566210589));
#42704=CARTESIAN_POINT('Ctrl Pts',(-0.819137482105158,-0.883185180518747,
59.7548817428246));
#42705=CARTESIAN_POINT('Ctrl Pts',(-0.658821672860672,-1.00844244930285,
59.7628068645903));
#42706=CARTESIAN_POINT('Ctrl Pts',(-0.478327079942962,-1.08780885724264,
59.770731986356));
#42707=CARTESIAN_POINT('Ctrl Pts',(-0.297832487025252,-1.16717526518242,
59.7786571081218));
#42708=CARTESIAN_POINT('Ctrl Pts',(-0.0971591104343092,-1.20065081227788,
59.7865822298875));
#42709=CARTESIAN_POINT('Ctrl Pts',(0.0993244585691621,-1.18417040430808,
59.7945073516532));
#42710=CARTESIAN_POINT('Ctrl Pts',(0.295808027572639,-1.16768999633827,
59.8024324734189));
#42711=CARTESIAN_POINT('Ctrl Pts',(0.488101788988651,-1.1012536333032,59.8103575951847));
#42712=CARTESIAN_POINT('Ctrl Pts',(0.652853226000178,-0.992928992641875,
59.8182827169504));
#42713=CARTESIAN_POINT('Ctrl Pts',(0.817604663011705,-0.88460435198055,
59.8262078387161));
#42714=CARTESIAN_POINT('Ctrl Pts',(0.954813775618739,-0.734391433692975,
59.8341329604818));
#42715=CARTESIAN_POINT('Ctrl Pts',(1.04782061281555,-0.56053185642523,59.8420580822475));
#42716=CARTESIAN_POINT('Ctrl Pts',(1.12495121150481,-0.416350055530902,
59.848630388165));
#42717=CARTESIAN_POINT('Ctrl Pts',(1.17168218150301,-0.255905525034767,
59.8552026940825));
#42718=CARTESIAN_POINT('Ctrl Pts',(1.18463057630128,-0.0928773270329352,
59.861775));
#42719=CARTESIAN_POINT('',(-0.590199102098993,-0.827621616530207,56.061775));
#42720=CARTESIAN_POINT('Ctrl Pts',(-0.590199102098968,-0.827621616530224,
56.061775));
#42721=CARTESIAN_POINT('Ctrl Pts',(-0.615134357767448,-0.812766705787686,
56.061775));
#42722=CARTESIAN_POINT('Ctrl Pts',(-0.639392267770691,-0.796859952851615,
56.061775));
#42723=CARTESIAN_POINT('Ctrl Pts',(-0.662901484824834,-0.779940878155282,
56.061775));
#42724=CARTESIAN_POINT('Ctrl Pts',(-0.698146337912065,-0.754575920204076,
56.061775));
#42725=CARTESIAN_POINT('Ctrl Pts',(-0.731709816296971,-0.726937622024356,
56.061775));
#42726=CARTESIAN_POINT('Ctrl Pts',(-0.763450748845136,-0.697254972180441,
56.061775));
#42727=CARTESIAN_POINT('Ctrl Pts',(-0.776265295565428,-0.685271401671611,
56.061775));
#42728=CARTESIAN_POINT('Ctrl Pts',(-0.788782535939489,-0.672954139864235,
56.061775));
#42729=CARTESIAN_POINT('Ctrl Pts',(-0.800992024443568,-0.660316467040226,
56.061775));
#42730=CARTESIAN_POINT('Ctrl Pts',(-0.808384981105688,-0.652664240866562,
56.061775));
#42731=CARTESIAN_POINT('Ctrl Pts',(-0.815659101518573,-0.644900665985542,
56.061775));
#42732=CARTESIAN_POINT('Ctrl Pts',(-0.822810165450187,-0.637031793761004,
56.061775));
#42733=CARTESIAN_POINT('Ctrl Pts',(-0.853515682503708,-0.603244123479613,
56.061775));
#42734=CARTESIAN_POINT('Ctrl Pts',(-0.881968856256046,-0.567503882812971,
56.061775));
#42735=CARTESIAN_POINT('Ctrl Pts',(-0.908008022156744,-0.530066595828932,
56.061775));
#42736=CARTESIAN_POINT('Ctrl Pts',(-0.924969563415267,-0.505680481073624,
56.061775));
#42737=CARTESIAN_POINT('Ctrl Pts',(-0.940906332635631,-0.480573325113094,
56.061775));
#42738=CARTESIAN_POINT('Ctrl Pts',(-0.955765822442545,-0.454806995938702,
56.061775));
#42739=CARTESIAN_POINT('Ctrl Pts',(-0.962684813681071,-0.442809477307636,
56.061775));
#42740=CARTESIAN_POINT('Ctrl Pts',(-0.969372662773929,-0.430663710074883,
56.061775));
#42741=CARTESIAN_POINT('Ctrl Pts',(-0.975808677947894,-0.418405110522661,
56.061775));
#42742=CARTESIAN_POINT('Ctrl Pts',(-0.981874487414775,-0.406851637262477,
56.061775));
#42743=CARTESIAN_POINT('Ctrl Pts',(-0.987719049555523,-0.39519409417799,
56.061775));
#42744=CARTESIAN_POINT('Ctrl Pts',(-0.993339017601775,-0.383438440842466,
56.061775));
#42745=CARTESIAN_POINT('Ctrl Pts',(-1.01324908218045,-0.341791261508261,
56.061775));
#42746=CARTESIAN_POINT('Ctrl Pts',(-1.03034352792734,-0.298915493303166,
56.061775));
#42747=CARTESIAN_POINT('Ctrl Pts',(-1.04462831590242,-0.255120180705625,
56.061775));
#42748=CARTESIAN_POINT('Ctrl Pts',(-1.05904170449985,-0.210930595230794,
56.061775));
#42749=CARTESIAN_POINT('Ctrl Pts',(-1.0705950057442,-0.165803798615469,
56.061775));
#42750=CARTESIAN_POINT('Ctrl Pts',(-1.07924869357493,-0.120029021709373,
56.061775));
#42751=CARTESIAN_POINT('Ctrl Pts',(-1.08423255818454,-0.0936662391480227,
56.061775));
#42752=CARTESIAN_POINT('Ctrl Pts',(-1.08825378413265,-0.0670880899307722,
56.061775));
#42753=CARTESIAN_POINT('Ctrl Pts',(-1.09129725999253,-0.0403477199554475,
56.061775));
#42754=CARTESIAN_POINT('Ctrl Pts',(-1.09228584736055,-0.0316618643118283,
56.061775));
#42755=CARTESIAN_POINT('Ctrl Pts',(-1.09317007591419,-0.0229689788750462,
56.061775));
#42756=CARTESIAN_POINT('Ctrl Pts',(-1.09394999532767,-0.014271318779927,
56.061775));
#42757=CARTESIAN_POINT('Ctrl Pts',(-1.09820214619636,0.0331486611431905,
56.061775));
#42758=CARTESIAN_POINT('Ctrl Pts',(-1.09935785012545,0.0807113437002552,
56.061775));
#42759=CARTESIAN_POINT('Ctrl Pts',(-1.09740239594642,0.128108944348922,
56.061775));
#42760=CARTESIAN_POINT('Ctrl Pts',(-1.0971991706204,0.133034855141317,56.061775));
#42761=CARTESIAN_POINT('Ctrl Pts',(-1.09696229903521,0.137959000314265,
56.061775));
#42762=CARTESIAN_POINT('Ctrl Pts',(-1.09669173443149,0.142881045058402,
56.061775));
#42763=CARTESIAN_POINT('Ctrl Pts',(-1.09412391271685,0.189594226312492,
56.061775));
#42764=CARTESIAN_POINT('Ctrl Pts',(-1.08852549990792,0.236117919595857,
56.061775));
#42765=CARTESIAN_POINT('Ctrl Pts',(-1.08001366796156,0.282192064001538,
56.061775));
#42766=CARTESIAN_POINT('Ctrl Pts',(-1.07595996531885,0.304134564994794,
56.061775));
#42767=CARTESIAN_POINT('Ctrl Pts',(-1.07124473547026,0.325975153615651,
56.061775));
#42768=CARTESIAN_POINT('Ctrl Pts',(-1.06587669291147,0.347685494908889,
56.061775));
#42769=CARTESIAN_POINT('Ctrl Pts',(-1.06298190770522,0.359393072505361,
56.061775));
#42770=CARTESIAN_POINT('Ctrl Pts',(-1.05989723894755,0.37106276652936,56.061775));
#42771=CARTESIAN_POINT('Ctrl Pts',(-1.05662375707351,0.3826900597016,56.061775));
#42772=CARTESIAN_POINT('Ctrl Pts',(-1.05399617734826,0.392023131022726,
56.061775));
#42773=CARTESIAN_POINT('Ctrl Pts',(-1.05124881344766,0.401321987665181,
56.061775));
#42774=CARTESIAN_POINT('Ctrl Pts',(-1.04838510858005,0.410577137809347,
56.061775));
#42775=CARTESIAN_POINT('Ctrl Pts',(-1.03397913167826,0.457135524711359,
56.061775));
#42776=CARTESIAN_POINT('Ctrl Pts',(-1.01661730418623,0.502644930856158,
56.061775));
#42777=CARTESIAN_POINT('Ctrl Pts',(-0.996446590099755,0.54682452658831,
56.061775));
#42778=CARTESIAN_POINT('Ctrl Pts',(-0.976533823419174,0.590439144201009,
56.061775));
#42779=CARTESIAN_POINT('Ctrl Pts',(-0.953883183691056,0.632758814049037,
56.061775));
#42780=CARTESIAN_POINT('Ctrl Pts',(-0.928586748315069,0.673506306109805,
56.061775));
#42781=CARTESIAN_POINT('Ctrl Pts',(-0.915799325391781,0.694104283899948,
56.061775));
#42782=CARTESIAN_POINT('Ctrl Pts',(-0.902335055056348,0.7143003027281,56.061775));
#42783=CARTESIAN_POINT('Ctrl Pts',(-0.888220713491049,0.734071072891337,
56.061775));
#42784=CARTESIAN_POINT('Ctrl Pts',(-0.879122478025178,0.746815494687745,
56.061775));
#42785=CARTESIAN_POINT('Ctrl Pts',(-0.869754065159863,0.759383184937614,
56.061775));
#42786=CARTESIAN_POINT('Ctrl Pts',(-0.860122058821546,0.771767493293035,
56.061775));
#42787=CARTESIAN_POINT('Ctrl Pts',(-0.854552989740373,0.778927898543135,
56.061775));
#42788=CARTESIAN_POINT('Ctrl Pts',(-0.848896461607506,0.786025972038092,
56.061775));
#42789=CARTESIAN_POINT('Ctrl Pts',(-0.843162068000595,0.793050710973022,
56.061775));
#42790=CARTESIAN_POINT('Ctrl Pts',(-0.811996437531328,0.831229188558734,
56.061775));
#42791=CARTESIAN_POINT('Ctrl Pts',(-0.778473601297604,0.867322786293068,
56.061775));
#42792=CARTESIAN_POINT('Ctrl Pts',(-0.742860732609996,0.901167302089467,
56.061775));
#42793=CARTESIAN_POINT('Ctrl Pts',(-0.706923922034914,0.935319674476243,
56.061775));
#42794=CARTESIAN_POINT('Ctrl Pts',(-0.668858204757825,0.967182723574884,
56.061775));
#42795=CARTESIAN_POINT('Ctrl Pts',(-0.628892453156465,0.996561433376393,
56.061775));
#42796=CARTESIAN_POINT('Ctrl Pts',(-0.591486565579768,1.02405839444809,
56.061775));
#42797=CARTESIAN_POINT('Ctrl Pts',(-0.552415331592047,1.04937941259432,
56.061775));
#42798=CARTESIAN_POINT('Ctrl Pts',(-0.511838811167469,1.07233375495117,
56.061775));
#42799=CARTESIAN_POINT('Ctrl Pts',(-0.590199102098993,-0.827621616530207,
56.061775));
#42800=CARTESIAN_POINT('Ctrl Pts',(-0.476210674841661,-0.908735228656824,
56.0683473059175));
#42801=CARTESIAN_POINT('Ctrl Pts',(-0.187550710949804,-1.03567600475847,
56.0828447336007));
#42802=CARTESIAN_POINT('Ctrl Pts',(0.304414618904077,-1.01477332192588,
56.1052672830496));
#42803=CARTESIAN_POINT('Ctrl Pts',(0.752129524692829,-0.746145432160931,
56.1290426483468));
#42804=CARTESIAN_POINT('Ctrl Pts',(1.01717154895307,-0.296300389836015,
56.1528180136439));
#42805=CARTESIAN_POINT('Ctrl Pts',(1.03517049480264,0.225508677645759,56.1765933789411));
#42806=CARTESIAN_POINT('Ctrl Pts',(0.801754274033107,0.69254746844306,56.2003687442382));
#42807=CARTESIAN_POINT('Ctrl Pts',(0.373613677358384,0.991385317760177,
56.2241441095354));
#42808=CARTESIAN_POINT('Ctrl Pts',(-0.14526763822163,1.04944237138876,56.2479194748325));
#42809=CARTESIAN_POINT('Ctrl Pts',(-0.628867346267627,0.852618234981034,
56.2716948401297));
#42810=CARTESIAN_POINT('Ctrl Pts',(-0.946309424739493,0.465101894360692,
56.2945056710427));
#42811=CARTESIAN_POINT('Ctrl Pts',(-1.0164049690006,0.148138950569523,56.30939138019));
#42812=CARTESIAN_POINT('Ctrl Pts',(-1.01653237544382,-1.90345246380841E-5,
56.3163519675715));
#42813=CARTESIAN_POINT('Origin',(-1.39932914042665E-16,0.,56.061775));
#42814=CARTESIAN_POINT('',(-1.188225,-1.45515594291686E-16,56.061775));
#42815=CARTESIAN_POINT('Origin',(0.,0.,56.061775));
#42816=CARTESIAN_POINT('Origin',(0.,0.,56.061775));
#42817=CARTESIAN_POINT('',(0.590159702139036,-0.827606761449038,56.061775));
#42818=CARTESIAN_POINT('Ctrl Pts',(0.51188116271663,1.07235883428022,56.061775));
#42819=CARTESIAN_POINT('Ctrl Pts',(0.541213176492396,1.05580342052956,56.061775));
#42820=CARTESIAN_POINT('Ctrl Pts',(0.569790684119403,1.03802023520366,56.061775));
#42821=CARTESIAN_POINT('Ctrl Pts',(0.597526191562895,1.01903462026179,56.061775));
#42822=CARTESIAN_POINT('Ctrl Pts',(0.637347544902611,0.991775956164436,
56.061775));
#42823=CARTESIAN_POINT('Ctrl Pts',(0.675434955264935,0.962039574884752,
56.061775));
#42824=CARTESIAN_POINT('Ctrl Pts',(0.71159321261738,0.93002723358959,56.061775));
#42825=CARTESIAN_POINT('Ctrl Pts',(0.726011613921828,0.917262050273659,
56.061775));
#42826=CARTESIAN_POINT('Ctrl Pts',(0.740122868411796,0.904134654496627,
56.061775));
#42827=CARTESIAN_POINT('Ctrl Pts',(0.753912893302178,0.890656748358753,
56.061775));
#42828=CARTESIAN_POINT('Ctrl Pts',(0.761733778079262,0.883012878838677,
56.061775));
#42829=CARTESIAN_POINT('Ctrl Pts',(0.769449908587933,0.875257488451145,
56.061775));
#42830=CARTESIAN_POINT('Ctrl Pts',(0.777050882853695,0.867401269087382,
56.061775));
#42831=CARTESIAN_POINT('Ctrl Pts',(0.811293653595113,0.832008606362631,
56.061775));
#42832=CARTESIAN_POINT('Ctrl Pts',(0.843249837994183,0.794526298977129,
56.061775));
#42833=CARTESIAN_POINT('Ctrl Pts',(0.872709194442015,0.755171056647391,
56.061775));
#42834=CARTESIAN_POINT('Ctrl Pts',(0.89231737439278,0.728976164203832,56.061775));
#42835=CARTESIAN_POINT('Ctrl Pts',(0.910818581336676,0.701950826308563,
56.061775));
#42836=CARTESIAN_POINT('Ctrl Pts',(0.928139018358984,0.674153489571596,
56.061775));
#42837=CARTESIAN_POINT('Ctrl Pts',(0.934162982461366,0.664485710494795,
56.061775));
#42838=CARTESIAN_POINT('Ctrl Pts',(0.940044027421705,0.654724521261419,
56.061775));
#42839=CARTESIAN_POINT('Ctrl Pts',(0.945778745449567,0.644872304782569,
56.061775));
#42840=CARTESIAN_POINT('Ctrl Pts',(0.950955710423823,0.635978305220254,
56.061775));
#42841=CARTESIAN_POINT('Ctrl Pts',(0.956008715846062,0.627018150888133,
56.061775));
#42842=CARTESIAN_POINT('Ctrl Pts',(0.96093425992874,0.617996981091859,56.061775));
#42843=CARTESIAN_POINT('Ctrl Pts',(0.966240504073969,0.608278556363322,
56.061775));
#42844=CARTESIAN_POINT('Ctrl Pts',(0.971399496552275,0.598488166785784,
56.061775));
#42845=CARTESIAN_POINT('Ctrl Pts',(0.976408975960127,0.588628330568485,
56.061775));
#42846=CARTESIAN_POINT('Ctrl Pts',(0.998306629291214,0.545528587499521,
56.061775));
#42847=CARTESIAN_POINT('Ctrl Pts',(1.01735139806086,0.501103250971285,56.061775));
#42848=CARTESIAN_POINT('Ctrl Pts',(1.03348950286457,0.455649362549699,56.061775));
#42849=CARTESIAN_POINT('Ctrl Pts',(1.04951099106991,0.410523931398352,56.061775));
#42850=CARTESIAN_POINT('Ctrl Pts',(1.06266777045703,0.364383618467088,56.061775));
#42851=CARTESIAN_POINT('Ctrl Pts',(1.07285691829592,0.317511905876643,56.061775));
#42852=CARTESIAN_POINT('Ctrl Pts',(1.07837716427354,0.292117889911543,56.061775));
#42853=CARTESIAN_POINT('Ctrl Pts',(1.08302546433836,0.266509169083111,56.061775));
#42854=CARTESIAN_POINT('Ctrl Pts',(1.08677904430391,0.240731714446861,56.061775));
#42855=CARTESIAN_POINT('Ctrl Pts',(1.0880860079379,0.231756230749861,56.061775));
#42856=CARTESIAN_POINT('Ctrl Pts',(1.08928435565178,0.222760175096169,56.061775));
#42857=CARTESIAN_POINT('Ctrl Pts',(1.09037158929866,0.213760065440079,56.061775));
#42858=CARTESIAN_POINT('Ctrl Pts',(1.09603301779298,0.166894814897787,56.061775));
#42859=CARTESIAN_POINT('Ctrl Pts',(1.09870084944373,0.119821996076729,56.061775));
#42860=CARTESIAN_POINT('Ctrl Pts',(1.09830409626352,0.0728155162236506,
56.061775));
#42861=CARTESIAN_POINT('Ctrl Pts',(1.09823697088453,0.0648626429196009,
56.061775));
#42862=CARTESIAN_POINT('Ctrl Pts',(1.09808200359928,0.0569116710356248,
56.061775));
#42863=CARTESIAN_POINT('Ctrl Pts',(1.09783870224064,0.0489639378119466,
56.061775));
#42864=CARTESIAN_POINT('Ctrl Pts',(1.09646708930469,0.00415854189393555,
56.061775));
#42865=CARTESIAN_POINT('Ctrl Pts',(1.09229131175929,-0.0405450829525213,
56.061775));
#42866=CARTESIAN_POINT('Ctrl Pts',(1.08536508685724,-0.0848917630206196,
56.061775));
#42867=CARTESIAN_POINT('Ctrl Pts',(1.08219399192013,-0.105195396620489,
56.061775));
#42868=CARTESIAN_POINT('Ctrl Pts',(1.07844580825791,-0.125424005149654,
56.061775));
#42869=CARTESIAN_POINT('Ctrl Pts',(1.0741230344062,-0.145551711443283,56.061775));
#42870=CARTESIAN_POINT('Ctrl Pts',(1.07095359998539,-0.16030923689511,56.061775));
#42871=CARTESIAN_POINT('Ctrl Pts',(1.06747524639181,-0.175012501031669,
56.061775));
#42872=CARTESIAN_POINT('Ctrl Pts',(1.0636884290732,-0.189650892812463,56.061775));
#42873=CARTESIAN_POINT('Ctrl Pts',(1.06147412044756,-0.198210565608511,
56.061775));
#42874=CARTESIAN_POINT('Ctrl Pts',(1.05915657217545,-0.206739316939933,
56.061775));
#42875=CARTESIAN_POINT('Ctrl Pts',(1.0567371423407,-0.215232892687751,56.061775));
#42876=CARTESIAN_POINT('Ctrl Pts',(1.04410920283738,-0.259564147585017,
56.061775));
#42877=CARTESIAN_POINT('Ctrl Pts',(1.02870411368939,-0.302960040082526,
56.061775));
#42878=CARTESIAN_POINT('Ctrl Pts',(1.01059776657305,-0.345147467590477,
56.061775));
#42879=CARTESIAN_POINT('Ctrl Pts',(0.993177632510785,-0.38573603237434,
56.061775));
#42880=CARTESIAN_POINT('Ctrl Pts',(0.973256491999253,-0.425206742761526,
56.061775));
#42881=CARTESIAN_POINT('Ctrl Pts',(0.950863549147145,-0.463291842602604,
56.061775));
#42882=CARTESIAN_POINT('Ctrl Pts',(0.939898284887777,-0.481941163813304,
56.061775));
#42883=CARTESIAN_POINT('Ctrl Pts',(0.928339758868041,-0.500257777247556,
56.061775));
#42884=CARTESIAN_POINT('Ctrl Pts',(0.916206631623963,-0.518216412717626,
56.061775));
#42885=CARTESIAN_POINT('Ctrl Pts',(0.906618806063435,-0.532407664546469,
56.061775));
#42886=CARTESIAN_POINT('Ctrl Pts',(0.896672138992213,-0.546375343126482,
56.061775));
#42887=CARTESIAN_POINT('Ctrl Pts',(0.886375271377727,-0.560105994464807,
56.061775));
#42888=CARTESIAN_POINT('Ctrl Pts',(0.881062189104107,-0.567190875320056,
56.061775));
#42889=CARTESIAN_POINT('Ctrl Pts',(0.875661590439594,-0.574204963613947,
56.061775));
#42890=CARTESIAN_POINT('Ctrl Pts',(0.870176513113682,-0.581145175673688,
56.061775));
#42891=CARTESIAN_POINT('Ctrl Pts',(0.842127545718367,-0.616635246316926,
56.061775));
#42892=CARTESIAN_POINT('Ctrl Pts',(0.81186116587577,-0.650211508350667,
56.061775));
#42893=CARTESIAN_POINT('Ctrl Pts',(0.779583315567684,-0.681676312373442,
56.061775));
#42894=CARTESIAN_POINT('Ctrl Pts',(0.747876545089263,-0.712584421487781,
56.061775));
#42895=CARTESIAN_POINT('Ctrl Pts',(0.714227917032577,-0.741455699548816,
56.061775));
#42896=CARTESIAN_POINT('Ctrl Pts',(0.678805048714601,-0.768062116484009,
56.061775));
#42897=CARTESIAN_POINT('Ctrl Pts',(0.650373815730447,-0.789417056800181,
56.061775));
#42898=CARTESIAN_POINT('Ctrl Pts',(0.620798928602909,-0.809312328764666,
56.061775));
#42899=CARTESIAN_POINT('Ctrl Pts',(0.590159702138998,-0.827606761449064,
56.061775));
#42900=CARTESIAN_POINT('Origin',(0.,0.,56.061775));
#42901=CARTESIAN_POINT('Origin',(0.,0.,55.5071980324285));
#42902=CARTESIAN_POINT('Ctrl Pts',(0.590159702138998,-0.827606761449064,
56.061775));
#42903=CARTESIAN_POINT('Ctrl Pts',(0.727528654917474,-0.729650069900356,
56.0697001217657));
#42904=CARTESIAN_POINT('Ctrl Pts',(0.952386591942655,-0.464074653132307,
56.0855503652972));
#42905=CARTESIAN_POINT('Ctrl Pts',(1.05840218504528,0.0472158302600112,
56.1093257305943));
#42906=CARTESIAN_POINT('Ctrl Pts',(0.907323368999851,0.546975187147921,
56.1331010958915));
#42907=CARTESIAN_POINT('Ctrl Pts',(0.535893220447681,0.913924938167876,
56.1568764611886));
#42908=CARTESIAN_POINT('Ctrl Pts',(0.0343021097832936,1.05889180686411,
56.1806518264858));
#42909=CARTESIAN_POINT('Ctrl Pts',(-0.475617027886791,0.946689808672358,
56.2044271917829));
#42910=CARTESIAN_POINT('Ctrl Pts',(-0.870023079724685,0.604559065518011,
56.22820255708));
#42911=CARTESIAN_POINT('Ctrl Pts',(-1.00549040154112,0.242800257196262,
56.2457928372953));
#42912=CARTESIAN_POINT('Ctrl Pts',(-1.01652086625353,0.0370683686476844,
56.2554579957447));
#42913=CARTESIAN_POINT('Ctrl Pts',(-1.01648283811887,2.60095369413633E-5,
56.2571980324285));
#42914=CARTESIAN_POINT('Ctrl Pts',(0.689876791927102,-0.967444397671189,
55.9626150912667));
#42915=CARTESIAN_POINT('Ctrl Pts',(0.850456465716625,-0.85293632829864,
55.9705402130324));
#42916=CARTESIAN_POINT('Ctrl Pts',(1.11330781200822,-0.542487621159544,
55.9863904565638));
#42917=CARTESIAN_POINT('Ctrl Pts',(1.2372364655554,0.0551937134810881,56.010165821861));
#42918=CARTESIAN_POINT('Ctrl Pts',(1.06063042389617,0.639395550061563,56.0339411871581));
#42919=CARTESIAN_POINT('Ctrl Pts',(0.626441104667066,1.06834743565215,56.0577165524553));
#42920=CARTESIAN_POINT('Ctrl Pts',(0.0400980096876628,1.23780881695182,
56.0814919177524));
#42921=CARTESIAN_POINT('Ctrl Pts',(-0.555980268044734,1.10664846445778,
56.1052672830496));
#42922=CARTESIAN_POINT('Ctrl Pts',(-1.01702764347953,0.706709162178262,
56.1290426483467));
#42923=CARTESIAN_POINT('Ctrl Pts',(-1.2310656854131,0.135131117029301,56.1528180136439));
#42924=CARTESIAN_POINT('Ctrl Pts',(-1.14611146910879,-0.469267475342316,
56.1765933789411));
#42925=CARTESIAN_POINT('Ctrl Pts',(-0.782797550539819,-0.959693272702349,
56.2003687442382));
#42926=CARTESIAN_POINT('Ctrl Pts',(-0.229363317643444,-1.21703566512132,
56.2241441095354));
#42927=CARTESIAN_POINT('Ctrl Pts',(0.379777109177097,-1.17879286552796,
56.2479194748325));
#42928=CARTESIAN_POINT('Ctrl Pts',(0.896679912107581,-0.854253141586999,
56.2716948401297));
#42929=CARTESIAN_POINT('Ctrl Pts',(1.19580337944822,-0.322238373221072,
56.2954702054269));
#42930=CARTESIAN_POINT('Ctrl Pts',(1.20449848491306,0.288039388201827,56.319245570724));
#42931=CARTESIAN_POINT('Ctrl Pts',(0.920653427402792,0.828360162236165,
56.3430209360211));
#42932=CARTESIAN_POINT('Ctrl Pts',(0.41320650609164,1.16749461393021,56.3667963013183));
#42933=CARTESIAN_POINT('Ctrl Pts',(-0.19459712002736,1.22307614310528,56.3905716666154));
#42934=CARTESIAN_POINT('Ctrl Pts',(-0.75513835931515,0.981605495597739,
56.4143470319126));
#42935=CARTESIAN_POINT('Ctrl Pts',(-1.13227687719907,0.501729373380553,
56.4381223972098));
#42936=CARTESIAN_POINT('Ctrl Pts',(-1.23441590924795,-0.100003268739267,
56.4618977625069));
#42937=CARTESIAN_POINT('Ctrl Pts',(-1.03674864192874,-0.677447816589128,
56.4856731278041));
#42938=CARTESIAN_POINT('Ctrl Pts',(-0.587283118157996,-1.09035857858026,
56.5094484931012));
#42939=CARTESIAN_POINT('Ctrl Pts',(0.00481762038262453,-1.23845067777583,
56.5332238583984));
#42940=CARTESIAN_POINT('Ctrl Pts',(0.595748288989899,-1.08575654127344,
56.5569992236955));
#42941=CARTESIAN_POINT('Ctrl Pts',(1.04198778136724,-0.669361452604685,
56.5807745889927));
#42942=CARTESIAN_POINT('Ctrl Pts',(1.23515657175416,-0.0903965375675185,
56.6045499542899));
#42943=CARTESIAN_POINT('Ctrl Pts',(1.12833917586245,0.510523256048042,56.628325319587));
#42944=CARTESIAN_POINT('Ctrl Pts',(0.747478655449841,0.987450733150073,
56.6521006848842));
#42945=CARTESIAN_POINT('Ctrl Pts',(0.185075748994057,1.22455308496042,56.6758760501813));
#42946=CARTESIAN_POINT('Ctrl Pts',(-0.422277060480572,1.16424455117628,
56.6996514154785));
#42947=CARTESIAN_POINT('Ctrl Pts',(-0.927070171999913,0.821172446529851,
56.7234267807756));
#42948=CARTESIAN_POINT('Ctrl Pts',(-1.20670296646235,0.278659723467029,
56.7472021460728));
#42949=CARTESIAN_POINT('Ctrl Pts',(-1.19326018722141,-0.331531923567072,
56.7709775113699));
#42950=CARTESIAN_POINT('Ctrl Pts',(-0.890006722445684,-0.861203416594047,
56.7947528766671));
#42951=CARTESIAN_POINT('Ctrl Pts',(-0.370594651923479,-1.18171184927523,
56.8185282419642));
#42952=CARTESIAN_POINT('Ctrl Pts',(0.238824854763645,-1.21521437594315,
56.8423036072614));
#42953=CARTESIAN_POINT('Ctrl Pts',(0.790240251682412,-0.953574137323725,
56.8660789725585));
#42954=CARTESIAN_POINT('Ctrl Pts',(1.14972762524983,-0.460336483986605,
56.8898543378557));
#42955=CARTESIAN_POINT('Ctrl Pts',(1.22997719735517,0.144704473801232,56.9136297031528));
#42956=CARTESIAN_POINT('Ctrl Pts',(1.01149851339784,0.714600621428312,56.93740506845));
#42957=CARTESIAN_POINT('Ctrl Pts',(0.547354147534323,1.11093956988161,56.9611804337472));
#42958=CARTESIAN_POINT('Ctrl Pts',(-0.0497277640765374,1.23746128837702,
56.9849557990443));
#42959=CARTESIAN_POINT('Ctrl Pts',(-0.634732144272647,1.0634370671454,57.0087311643415));
#42960=CARTESIAN_POINT('Ctrl Pts',(-1.06557722222055,0.631132691465518,
57.0325065296386));
#42961=CARTESIAN_POINT('Ctrl Pts',(-1.23762235982929,0.0455432234513654,
57.0562818949358));
#42962=CARTESIAN_POINT('Ctrl Pts',(-1.10908243780363,-0.551107464027959,
57.0800572602329));
#42963=CARTESIAN_POINT('Ctrl Pts',(-0.711176333065604,-1.01390902651033,
57.1038326255301));
#42964=CARTESIAN_POINT('Ctrl Pts',(-0.140544696353038,-1.2304594585271,
57.1276079908272));
#42965=CARTESIAN_POINT('Ctrl Pts',(0.46422145287787,-1.14816450626194,57.1513833561244));
#42966=CARTESIAN_POINT('Ctrl Pts',(0.956240743595242,-0.787011391937999,
57.1751587214215));
#42967=CARTESIAN_POINT('Ctrl Pts',(1.21601497292081,-0.234714457126464,
57.1989340867187));
#42968=CARTESIAN_POINT('Ctrl Pts',(1.18045199356654,0.374588282834027,57.2227094520159));
#42969=CARTESIAN_POINT('Ctrl Pts',(0.858189093138855,0.892913641495793,
57.246484817313));
#42970=CARTESIAN_POINT('Ctrl Pts',(0.327495230156222,1.19437438225068,57.2702601826101));
#42971=CARTESIAN_POINT('Ctrl Pts',(-0.282738382980947,1.20575382957762,
57.2940355479073));
#42972=CARTESIAN_POINT('Ctrl Pts',(-0.824302475860749,0.924288222927029,
57.3178109132045));
#42973=CARTESIAN_POINT('Ctrl Pts',(-1.16566575069977,0.418337959546242,
57.3415862785016));
#42974=CARTESIAN_POINT('Ctrl Pts',(-1.22392028367976,-0.189215300515123,
57.3653616437988));
#42975=CARTESIAN_POINT('Ctrl Pts',(-0.984917621412899,-0.750813272246919,
57.3891370090959));
#42976=CARTESIAN_POINT('Ctrl Pts',(-0.506705058309881,-1.13005896953874,
57.4129123743931));
#42977=CARTESIAN_POINT('Ctrl Pts',(0.0945724841541603,-1.2348438508543,
57.4366877396902));
#42978=CARTESIAN_POINT('Ctrl Pts',(0.672880923350564,-1.03971849735525,
57.4604631049874));
#42979=CARTESIAN_POINT('Ctrl Pts',(1.0877647517472,-0.592073589689751,57.4842384702846));
#42980=CARTESIAN_POINT('Ctrl Pts',(1.23845988787003,-0.0006299910492471,
57.5080138355817));
#42981=CARTESIAN_POINT('Ctrl Pts',(1.08836655140774,0.59096661540952,57.5317892008789));
#42982=CARTESIAN_POINT('Ctrl Pts',(0.673938361780622,1.03903338506143,57.555564566176));
#42983=CARTESIAN_POINT('Ctrl Pts',(0.095828738106295,1.23474699582737,57.5793399314732));
#42984=CARTESIAN_POINT('Ctrl Pts',(-0.505555099006082,1.13057389524998,
57.6031152967703));
#42985=CARTESIAN_POINT('Ctrl Pts',(-0.984153250827362,0.751814917142313,
57.6268906620675));
#42986=CARTESIAN_POINT('Ctrl Pts',(-1.22372714679232,0.190460392090562,
57.6506660273646));
#42987=CARTESIAN_POINT('Ctrl Pts',(-1.16609075524636,-0.417151820421223,
57.6744413926618));
#42988=CARTESIAN_POINT('Ctrl Pts',(-0.82524239971067,-0.923449117424206,
57.6982167579589));
#42989=CARTESIAN_POINT('Ctrl Pts',(-0.283964944005771,-1.20546555377064,
57.7219921232561));
#42990=CARTESIAN_POINT('Ctrl Pts',(0.326279930516472,-1.19470695055061,
57.7457674885532));
#42991=CARTESIAN_POINT('Ctrl Pts',(0.857280218357737,-0.893786282040778,
57.7695428538504));
#42992=CARTESIAN_POINT('Ctrl Pts',(1.18007028479188,-0.375789054794004,
57.7933182191476));
#42993=CARTESIAN_POINT('Ctrl Pts',(1.21625313690915,0.233477188843838,57.8170935844447));
#42994=CARTESIAN_POINT('Ctrl Pts',(0.957040936743427,0.786038126396572,
57.8408689497418));
#42995=CARTESIAN_POINT('Ctrl Pts',(0.465389329872678,1.14769162338689,57.864644315039));
#42996=CARTESIAN_POINT('Ctrl Pts',(-0.139292781304968,1.23060180880254,
57.8884196803362));
#42997=CARTESIAN_POINT('Ctrl Pts',(-0.710144436332023,1.01463203689734,
57.9121950456333));
#42998=CARTESIAN_POINT('Ctrl Pts',(-1.10852117924344,0.552235534822328,
57.9359704109305));
#42999=CARTESIAN_POINT('Ctrl Pts',(-1.2376680539947,-0.0442840701915317,
57.9597457762276));
#43000=CARTESIAN_POINT('Ctrl Pts',(-1.06621877123237,-0.630048270074204,
57.9835211415248));
#43001=CARTESIAN_POINT('Ctrl Pts',(-0.635813733195539,-1.0627907543029,
58.007296506822));
#43002=CARTESIAN_POINT('Ctrl Pts',(-0.0509867041603225,-1.23741005602453,
58.0310718721191));
#43003=CARTESIAN_POINT('Ctrl Pts',(0.546223618848922,-1.11149586097446,
58.0548472374163));
#43004=CARTESIAN_POINT('Ctrl Pts',(1.0107709710081,-0.715629327877998,58.0786226027134));
#43005=CARTESIAN_POINT('Ctrl Pts',(1.2298293416664,-0.145955750582684,58.1023979680106));
#43006=CARTESIAN_POINT('Ctrl Pts',(1.15019536641724,0.459166538223408,58.1261733333077));
#43007=CARTESIAN_POINT('Ctrl Pts',(0.791209988003854,0.952769670820134,
58.1499486986049));
#43008=CARTESIAN_POINT('Ctrl Pts',(0.240061063466199,1.21497077189505,58.173724063902));
#43009=CARTESIAN_POINT('Ctrl Pts',(-0.36939221256026,1.18208827252943,58.1974994291992));
#43010=CARTESIAN_POINT('Ctrl Pts',(-0.889130092481378,0.862108444104235,
58.2212747944963));
#43011=CARTESIAN_POINT('Ctrl Pts',(-1.19292227640834,0.332745748583669,
58.2450501597935));
#43012=CARTESIAN_POINT('Ctrl Pts',(-1.20698584421457,-0.277431906271434,
58.2688255250906));
#43013=CARTESIAN_POINT('Ctrl Pts',(-0.927905134948138,-0.820228840805201,
58.2926008903878));
#43014=CARTESIAN_POINT('Ctrl Pts',(-0.423461318665824,-1.16381433327897,
58.316376255685));
#43015=CARTESIAN_POINT('Ctrl Pts',(0.183829819914051,-1.22474074320329,
58.3401516209821));
#43016=CARTESIAN_POINT('Ctrl Pts',(0.746473658012812,-0.98821069041209,
58.3639269862793));
#43017=CARTESIAN_POINT('Ctrl Pts',(1.12781919681433,-0.511670939226426,
58.3877023515764));
#43018=CARTESIAN_POINT('Ctrl Pts',(1.23524789996815,0.0891398697331011,
58.4114777168736));
#43019=CARTESIAN_POINT('Ctrl Pts',(1.04266823568555,0.668301010805869,58.4352530821707));
#43020=CARTESIAN_POINT('Ctrl Pts',(0.596852605428911,1.08514987819401,58.4590284474679));
#43021=CARTESIAN_POINT('Ctrl Pts',(0.00607759029129267,1.23844513550178,
58.4828038127651));
#43022=CARTESIAN_POINT('Ctrl Pts',(-0.586173507453946,1.09095550317642,
58.5065791780622));
#43023=CARTESIAN_POINT('Ctrl Pts',(-1.03605888491723,0.678502231194445,
58.5303545433593));
#43024=CARTESIAN_POINT('Ctrl Pts',(-1.23431352927824,0.101259084493505,
58.5541299086565));
#43025=CARTESIAN_POINT('Ctrl Pts',(-1.13278673961859,-0.50057716018217,
58.5779052739537));
#43026=CARTESIAN_POINT('Ctrl Pts',(-0.756136632270754,-0.980836726519766,
58.6016806392508));
#43027=CARTESIAN_POINT('Ctrl Pts',(-0.195841350045654,-1.22287753122055,
58.625456004548));
#43028=CARTESIAN_POINT('Ctrl Pts',(0.412018509059322,-1.16791439709608,
58.6492313698451));
#43029=CARTESIAN_POINT('Ctrl Pts',(0.919810195403461,-0.829296385608678,
58.6730067351423));
#43030=CARTESIAN_POINT('Ctrl Pts',(1.20420481701146,-0.289264670221184,
58.6967821004394));
#43031=CARTESIAN_POINT('Ctrl Pts',(1.19613059797621,0.321021624406906,58.7205574657366));
#43032=CARTESIAN_POINT('Ctrl Pts',(0.897548548125092,0.853340432951767,
58.7443328310338));
#43033=CARTESIAN_POINT('Ctrl Pts',(0.380976186673455,1.17840588760389,58.7681081963309));
#43034=CARTESIAN_POINT('Ctrl Pts',(-0.228125005467955,1.21726836508307,
58.7918835616281));
#43035=CARTESIAN_POINT('Ctrl Pts',(-0.781820792375621,0.960489218763501,
58.8156589269252));
#43036=CARTESIAN_POINT('Ctrl Pts',(-1.14563341530098,0.47043317112805,58.8394342922223));
#43037=CARTESIAN_POINT('Ctrl Pts',(-1.23120260983117,-0.133878393688783,
58.8632096575195));
#43038=CARTESIAN_POINT('Ctrl Pts',(-1.01774592869022,-0.705674510937058,
58.8869850228167));
#43039=CARTESIAN_POINT('Ctrl Pts',(-0.557106237127393,-1.10608134027545,
58.9107603881138));
#43040=CARTESIAN_POINT('Ctrl Pts',(0.0388395194718907,-1.2378508724717,
58.934535753411));
#43041=CARTESIAN_POINT('Ctrl Pts',(0.62535220532555,-1.06897984548177,58.9583111187081));
#43042=CARTESIAN_POINT('Ctrl Pts',(1.059983722875,-0.64048247282172,58.9820864840053));
#43043=CARTESIAN_POINT('Ctrl Pts',(1.23717381007099,-0.056429198348077,
59.0058618493025));
#43044=CARTESIAN_POINT('Ctrl Pts',(1.11388777825955,0.541329205009086,59.0296372145996));
#43045=CARTESIAN_POINT('Ctrl Pts',(0.720068476266758,1.00761335850545,59.0534125798967));
#43046=CARTESIAN_POINT('Ctrl Pts',(0.151363980773296,1.22917542933311,59.0771879451939));
#43047=CARTESIAN_POINT('Ctrl Pts',(-0.454102739340545,1.15220397190566,
59.100963310491));
#43048=CARTESIAN_POINT('Ctrl Pts',(-0.949280163288418,0.795393275266316,
59.1247386757882));
#43049=CARTESIAN_POINT('Ctrl Pts',(-1.21390306288918,0.245403024961089,
59.1485140410854));
#43050=CARTESIAN_POINT('Ctrl Pts',(-1.18370167974241,-0.364188995065361,
59.1722894063825));
#43051=CARTESIAN_POINT('Ctrl Pts',(-0.866011114480599,-0.885329340046922,
59.1960647716797));
#43052=CARTESIAN_POINT('Ctrl Pts',(-0.337989828847549,-1.19144708919335,
59.2198401369768));
#43053=CARTESIAN_POINT('Ctrl Pts',(0.272120061643497,-1.20819450536858,
59.243615502274));
#43054=CARTESIAN_POINT('Ctrl Pts',(0.816139335472622,-0.931504093306501,
59.2673908675711));
#43055=CARTESIAN_POINT('Ctrl Pts',(1.16194039768241,-0.428576484402961,
59.2911662328683));
#43056=CARTESIAN_POINT('Ctrl Pts',(1.22553750571355,0.178440782463945,59.3149415981654));
#43057=CARTESIAN_POINT('Ctrl Pts',(0.991484638916142,0.742119600560311,
59.3387169634626));
#43058=CARTESIAN_POINT('Ctrl Pts',(0.516626920037774,1.12555760237105,59.3624923287597));
#43059=CARTESIAN_POINT('Ctrl Pts',(-0.0837055306015586,1.23562804876679,
59.3862676940569));
#43060=CARTESIAN_POINT('Ctrl Pts',(-0.66370816752893,1.04559779985052,59.4100430593541));
#43061=CARTESIAN_POINT('Ctrl Pts',(-1.08251400861023,0.601620072902204,
59.4338184246512));
#43062=CARTESIAN_POINT('Ctrl Pts',(-1.23840642074766,0.011525071951662,
59.4575937899484));
#43063=CARTESIAN_POINT('Ctrl Pts',(-1.0935233469385,-0.581369057887385,
59.4813691552455));
#43064=CARTESIAN_POINT('Ctrl Pts',(-0.683052971567649,-1.033064338435,59.5051445205427));
#43065=CARTESIAN_POINT('Ctrl Pts',(-0.106687473759109,-1.23385618060568,
59.5289198858398));
#43066=CARTESIAN_POINT('Ctrl Pts',(0.495589540417238,-1.13497766591134,
59.552695251137));
#43067=CARTESIAN_POINT('Ctrl Pts',(0.977501214644604,-0.760443717735149,
59.5764706164341));
#43068=CARTESIAN_POINT('Ctrl Pts',(1.22200427569806,-0.201218517620435,
59.6002459817313));
#43069=CARTESIAN_POINT('Ctrl Pts',(1.16971539613015,0.406877223320946,59.6240213470285));
#43070=CARTESIAN_POINT('Ctrl Pts',(0.83333442333768,0.916153481637932,59.6477967123256));
#43071=CARTESIAN_POINT('Ctrl Pts',(0.294558588880807,1.20292076975491,59.6715720776228));
#43072=CARTESIAN_POINT('Ctrl Pts',(-0.315756654949849,1.19753112793076,
59.6953474429199));
#43073=CARTESIAN_POINT('Ctrl Pts',(-0.849385120103183,0.901293403997361,
59.7191228082171));
#43074=CARTESIAN_POINT('Ctrl Pts',(-1.17671661268543,0.386156096850363,
59.7428981735142));
#43075=CARTESIAN_POINT('Ctrl Pts',(-1.21826471063664,-0.222768480037991,
59.7666735388113));
#43076=CARTESIAN_POINT('Ctrl Pts',(-0.963909730368294,-0.777587035150415,
59.7904489041086));
#43077=CARTESIAN_POINT('Ctrl Pts',(-0.475491739768952,-1.14355062114423,
59.8142242694057));
#43078=CARTESIAN_POINT('Ctrl Pts',(0.128495139722361,-1.23176138211002,
59.8379996347029));
#43079=CARTESIAN_POINT('Ctrl Pts',(0.5101794029784,-1.09109740948615,59.8538498782343));
#43080=CARTESIAN_POINT('Ctrl Pts',(0.672748867539255,-0.97943229058963,
59.861775));
#43081=CARTESIAN_POINT('Ctrl Pts',(0.656637761997734,-0.920831852263814,
55.9956683941778));
#43082=CARTESIAN_POINT('Ctrl Pts',(0.809480528783575,-0.811840908832545,
56.0035935159435));
#43083=CARTESIAN_POINT('Ctrl Pts',(1.0596674053197,-0.516349965150465,56.0194437594749));
#43084=CARTESIAN_POINT('Ctrl Pts',(1.17762503871869,0.0525344190740624,
56.0432191247721));
#43085=CARTESIAN_POINT('Ctrl Pts',(1.00952807226406,0.608588762423683,56.0669944900692));
#43086=CARTESIAN_POINT('Ctrl Pts',(0.596258476593938,1.01687326982406,56.0907698553664));
#43087=CARTESIAN_POINT('Ctrl Pts',(0.0381660430528731,1.17816981358925,
56.1145452206636));
#43088=CARTESIAN_POINT('Ctrl Pts',(-0.529192521325419,1.0533289125293,56.1383205859607));
#43089=CARTESIAN_POINT('Ctrl Pts',(-0.968026122227916,0.672659129958179,
56.1620959512579));
#43090=CARTESIAN_POINT('Ctrl Pts',(-1.17175157361617,0.128620349750434,
56.185871316555));
#43091=CARTESIAN_POINT('Ctrl Pts',(-1.09089054579335,-0.44665764726822,
56.2096466818522));
#43092=CARTESIAN_POINT('Ctrl Pts',(-0.745081495273847,-0.913454185103445,
56.2334220471493));
#43093=CARTESIAN_POINT('Ctrl Pts',(-0.218312338296022,-1.15839753528211,
56.2571974124465));
#43094=CARTESIAN_POINT('Ctrl Pts',(0.361479026322095,-1.12199731624102,
56.2809727777436));
#43095=CARTESIAN_POINT('Ctrl Pts',(0.853476878197205,-0.813094276594377,
56.3047481430408));
#43096=CARTESIAN_POINT('Ctrl Pts',(1.13818824471077,-0.306712570560035,
56.3285235083379));
#43097=CARTESIAN_POINT('Ctrl Pts',(1.14646441033857,0.274161330616311,56.3522988736351));
#43098=CARTESIAN_POINT('Ctrl Pts',(0.876295322903381,0.788448849742304,
56.3760742389322));
#43099=CARTESIAN_POINT('Ctrl Pts',(0.393297757770615,1.11124342695173,56.3998496042294));
#43100=CARTESIAN_POINT('Ctrl Pts',(-0.185221214688251,1.16414697632897,
56.4236249695266));
#43101=CARTESIAN_POINT('Ctrl Pts',(-0.718754954597366,0.934310652766648,
56.4474003348237));
#43102=CARTESIAN_POINT('Ctrl Pts',(-1.07772251988488,0.477555495010681,
56.4711757001209));
#43103=CARTESIAN_POINT('Ctrl Pts',(-1.17494037994631,-0.0951850001997911,
56.494951065418));
#43104=CARTESIAN_POINT('Ctrl Pts',(-0.986796941072066,-0.644807628493671,
56.5187264307152));
#43105=CARTESIAN_POINT('Ctrl Pts',(-0.558987165359032,-1.03782389144296,
56.5425017960123));
#43106=CARTESIAN_POINT('Ctrl Pts',(0.00458550208272216,-1.17878074884598,
56.5662771613095));
#43107=CARTESIAN_POINT('Ctrl Pts',(0.567044474859859,-1.03344358540405,
56.5900525266066));
#43108=CARTESIAN_POINT('Ctrl Pts',(0.991783652954465,-0.637110874505737,
56.6138278919038));
#43109=CARTESIAN_POINT('Ctrl Pts',(1.17564535651048,-0.0860411320039726,
56.637603257201));
#43110=CARTESIAN_POINT('Ctrl Pts',(1.0739745413714,0.485925678645828,56.6613786224981));
#43111=CARTESIAN_POINT('Ctrl Pts',(0.711464303770228,0.939874260282695,
56.6851539877953));
#43112=CARTESIAN_POINT('Ctrl Pts',(0.176158593884617,1.16555275748542,56.7089293530924));
#43113=CARTESIAN_POINT('Ctrl Pts',(-0.401931282776427,1.10814995583041,
56.7327047183896));
#43114=CARTESIAN_POINT('Ctrl Pts',(-0.882402901620151,0.78160744616053,
56.7564800836867));
#43115=CARTESIAN_POINT('Ctrl Pts',(-1.14856267751879,0.265233588544357,
56.7802554489839));
#43116=CARTESIAN_POINT('Ctrl Pts',(-1.13576758630961,-0.31555834733007,
56.804030814281));
#43117=CARTESIAN_POINT('Ctrl Pts',(-0.847125210223656,-0.81970967963345,
56.8278061795782));
#43118=CARTESIAN_POINT('Ctrl Pts',(-0.352738990055884,-1.12477566010987,
56.8515815448753));
#43119=CARTESIAN_POINT('Ctrl Pts',(0.227318008050931,-1.15666399783905,
56.8753569101725));
#43120=CARTESIAN_POINT('Ctrl Pts',(0.752165598810427,-0.907629876462535,
56.8991322754696));
#43121=CARTESIAN_POINT('Ctrl Pts',(1.09433247151586,-0.438156960993706,
56.9229076407668));
#43122=CARTESIAN_POINT('Ctrl Pts',(1.17071553012162,0.137732451562079,56.946683006064));
#43123=CARTESIAN_POINT('Ctrl Pts',(0.962763391773544,0.68017036993826,56.9704583713611));
#43124=CARTESIAN_POINT('Ctrl Pts',(0.520982016880328,1.05741326772864,56.9942337366582));
#43125=CARTESIAN_POINT('Ctrl Pts',(-0.04733182518165,1.17783902932711,57.0180091019554));
#43126=CARTESIAN_POINT('Ctrl Pts',(-0.604150044704295,1.01219948832483,
57.0417844672526));
#43127=CARTESIAN_POINT('Ctrl Pts',(-1.01423652835186,0.600724017530526,
57.0655598325497));
#43128=CARTESIAN_POINT('Ctrl Pts',(-1.17799234017794,0.0433489003706404,
57.0893351978469));
#43129=CARTESIAN_POINT('Ctrl Pts',(-1.05564561433647,-0.524554494417324,
57.113110563144));
#43130=CARTESIAN_POINT('Ctrl Pts',(-0.676911067591465,-0.965057763687454,
57.1368859284412));
#43131=CARTESIAN_POINT('Ctrl Pts',(-0.133773096810682,-1.17117455541475,
57.1606612937383));
#43132=CARTESIAN_POINT('Ctrl Pts',(0.441854747769617,-1.09284466533661,
57.1844366590355));
#43133=CARTESIAN_POINT('Ctrl Pts',(0.910168002682683,-0.749092309114078,
57.2082120243326));
#43134=CARTESIAN_POINT('Ctrl Pts',(1.15742602116528,-0.223405653936416,
57.2319873896298));
#43135=CARTESIAN_POINT('Ctrl Pts',(1.12357650564827,0.356540203394322,57.2557627549269));
#43136=CARTESIAN_POINT('Ctrl Pts',(0.816840589629669,0.849892070685862,
57.2795381202241));
#43137=CARTESIAN_POINT('Ctrl Pts',(0.311716146290415,1.13682809818508,57.3033134855212));
#43138=CARTESIAN_POINT('Ctrl Pts',(-0.269115733713632,1.14765927110315,
57.3270888508185));
#43139=CARTESIAN_POINT('Ctrl Pts',(-0.784586667202436,0.879754989942892,
57.3508642161156));
#43140=CARTESIAN_POINT('Ctrl Pts',(-1.10950268038265,0.398181972099398,
57.3746395814127));
#43141=CARTESIAN_POINT('Ctrl Pts',(-1.16495044527317,-0.180098697216517,
57.3984149467099));
#43142=CARTESIAN_POINT('Ctrl Pts',(-0.937463196681984,-0.714638255027005,
57.422190312007));
#43143=CARTESIAN_POINT('Ctrl Pts',(-0.482291445914716,-1.07561147347857,
57.4459656773042));
#43144=CARTESIAN_POINT('Ctrl Pts',(0.0900158768467722,-1.17534770285084,
57.4697410426014));
#43145=CARTESIAN_POINT('Ctrl Pts',(0.640460773242784,-0.989623705566161,
57.4935164078985));
#43146=CARTESIAN_POINT('Ctrl Pts',(1.03535503806711,-0.563546826652665,
57.5172917731957));
#43147=CARTESIAN_POINT('Ctrl Pts',(1.17878951518762,-0.000599637380898037,
57.5410671384928));
#43148=CARTESIAN_POINT('Ctrl Pts',(1.03592784235172,0.562493187622534,57.56484250379));
#43149=CARTESIAN_POINT('Ctrl Pts',(0.641467263115012,0.988971602743467,
57.5886178690871));
#43150=CARTESIAN_POINT('Ctrl Pts',(0.0912116030884411,1.17525551440667,
57.6123932343843));
#43151=CARTESIAN_POINT('Ctrl Pts',(-0.481196892927188,1.07610158949723,
57.6361685996814));
#43152=CARTESIAN_POINT('Ctrl Pts',(-0.936735654320081,0.715591639559026,
57.6599439649786));
#43153=CARTESIAN_POINT('Ctrl Pts',(-1.16476661393545,0.181283798897194,
57.6837193302757));
#43154=CARTESIAN_POINT('Ctrl Pts',(-1.10990720773822,-0.397052982474613,
57.7074946955729));
#43155=CARTESIAN_POINT('Ctrl Pts',(-0.785481304477495,-0.87895631347501,
57.73127006087));
#43156=CARTESIAN_POINT('Ctrl Pts',(-0.270283197666202,-1.14738488474469,
57.7550454261672));
#43157=CARTESIAN_POINT('Ctrl Pts',(0.310559401136881,-1.137144642975,57.7788207914644));
#43158=CARTESIAN_POINT('Ctrl Pts',(0.815975505444798,-0.850722666440334,
57.8025961567615));
#43159=CARTESIAN_POINT('Ctrl Pts',(1.12321318802626,-0.357683120827827,
57.8263715220587));
#43160=CARTESIAN_POINT('Ctrl Pts',(1.15765271014818,0.222227998613616,57.8501468873558));
#43161=CARTESIAN_POINT('Ctrl Pts',(0.910929641636386,0.748165936587234,
57.873922252653));
#43162=CARTESIAN_POINT('Ctrl Pts',(0.442966355153904,1.09239456648361,57.8976976179501));
#43163=CARTESIAN_POINT('Ctrl Pts',(-0.132581500419862,1.17131004709584,
57.9214729832473));
#43164=CARTESIAN_POINT('Ctrl Pts',(-0.675928888788414,0.965745938631122,
57.9452483485444));
#43165=CARTESIAN_POINT('Ctrl Pts',(-1.05511139783698,0.525628213508114,
57.9690237138416));
#43166=CARTESIAN_POINT('Ctrl Pts',(-1.17803583274772,-0.0421504145131365,
57.9927990791388));
#43167=CARTESIAN_POINT('Ctrl Pts',(-1.01484716681986,-0.599691844766081,
58.0165744444359));
#43168=CARTESIAN_POINT('Ctrl Pts',(-0.605179521471793,-1.0115843155528,
58.0403498097331));
#43169=CARTESIAN_POINT('Ctrl Pts',(-0.0485301081341635,-1.17779026540625,
58.0641251750302));
#43170=CARTESIAN_POINT('Ctrl Pts',(0.519905958322425,-1.05794275609888,
58.0879005403274));
#43171=CARTESIAN_POINT('Ctrl Pts',(0.962070903184065,-0.681149512168836,
58.1116759056245));
#43172=CARTESIAN_POINT('Ctrl Pts',(1.17057479828413,-0.138923440438677,
58.1354512709216));
#43173=CARTESIAN_POINT('Ctrl Pts',(1.0947776763944,0.437043384516588,58.1592266362188));
#43174=CARTESIAN_POINT('Ctrl Pts',(0.753088612159024,0.906864170048437,
58.183002001516));
#43175=CARTESIAN_POINT('Ctrl Pts',(0.228494654845404,1.1564321309045,58.2067773668131));
#43176=CARTESIAN_POINT('Ctrl Pts',(-0.351594485556477,1.12513394687367,
58.2305527321103));
#43177=CARTESIAN_POINT('Ctrl Pts',(-0.846290817264516,0.820571101913176,
58.2543280974074));
#43178=CARTESIAN_POINT('Ctrl Pts',(-1.13544595641476,0.316713688909432,
58.2781034627046));
#43179=CARTESIAN_POINT('Ctrl Pts',(-1.14883192590677,-0.26406492894472,
58.3018788280017));
#43180=CARTESIAN_POINT('Ctrl Pts',(-0.883197635126317,-0.780709304407554,
58.3256541932989));
#43181=CARTESIAN_POINT('Ctrl Pts',(-0.403058482087211,-1.10774046630914,
58.3494295585961));
#43182=CARTESIAN_POINT('Ctrl Pts',(0.174972695051272,-1.16573137414575,
58.3732049238932));
#43183=CARTESIAN_POINT('Ctrl Pts',(0.710507728225752,-0.940597601959907,
58.3969802891904));
#43184=CARTESIAN_POINT('Ctrl Pts',(1.07347961549125,-0.487018065174191,
58.4207556544875));
#43185=CARTESIAN_POINT('Ctrl Pts',(1.1757322844297,0.0848450118213287,58.4445310197847));
#43186=CARTESIAN_POINT('Ctrl Pts',(0.992431322228083,0.636101525970394,
58.4683063850818));
#43187=CARTESIAN_POINT('Ctrl Pts',(0.568095584106511,1.03286615202548,58.492081750379));
#43188=CARTESIAN_POINT('Ctrl Pts',(0.00578476524201244,1.17877547360485,
58.5158571156761));
#43189=CARTESIAN_POINT('Ctrl Pts',(-0.557931016930909,1.0383920555492,58.5396324809733));
#43190=CARTESIAN_POINT('Ctrl Pts',(-0.986140417319333,0.645811240232391,
58.5634078462705));
#43191=CARTESIAN_POINT('Ctrl Pts',(-1.17484293275723,0.0963803093564249,
58.5871832115676));
#43192=CARTESIAN_POINT('Ctrl Pts',(-1.07820781656684,-0.476458796723713,
58.6109585768648));
#43193=CARTESIAN_POINT('Ctrl Pts',(-0.719705129653402,-0.933578923836559,
58.6347339421619));
#43194=CARTESIAN_POINT('Ctrl Pts',(-0.186405496322565,-1.1639579337854,
58.6585093074591));
#43195=CARTESIAN_POINT('Ctrl Pts',(0.392166999754567,-1.11164298449851,
58.6822846727562));
#43196=CARTESIAN_POINT('Ctrl Pts',(0.875492718758175,-0.789339964833067,
58.7060600380534));
#43197=CARTESIAN_POINT('Ctrl Pts',(1.14618489168258,-0.275327577187317,
58.7298354033505));
#43198=CARTESIAN_POINT('Ctrl Pts',(1.13849969748671,0.305554446054918,58.7536107686477));
#43199=CARTESIAN_POINT('Ctrl Pts',(0.854303662366784,0.81222554327474,58.7773861339448));
#43200=CARTESIAN_POINT('Ctrl Pts',(0.362620330933121,1.12162898334307,58.801161499242));
#43201=CARTESIAN_POINT('Ctrl Pts',(-0.217133689376275,1.15861902350129,
58.8249368645392));
#43202=CARTESIAN_POINT('Ctrl Pts',(-0.744151798402677,0.914211781599485,
58.8487122298363));
#43203=CARTESIAN_POINT('Ctrl Pts',(-1.09043552514888,0.447767178536508,
58.8724875951335));
#43204=CARTESIAN_POINT('Ctrl Pts',(-1.17188190086373,-0.127427984011593,
58.8962629604306));
#43205=CARTESIAN_POINT('Ctrl Pts',(-0.968709799659506,-0.671674329362741,
58.9200383257278));
#43206=CARTESIAN_POINT('Ctrl Pts',(-0.530264239967304,-1.05278911301986,
58.9438136910249));
#43207=CARTESIAN_POINT('Ctrl Pts',(0.036968188293232,-1.17820984282748,
58.9675890563221));
#43208=CARTESIAN_POINT('Ctrl Pts',(0.595222041631902,-1.01747520944581,
58.9913644216192));
#43209=CARTESIAN_POINT('Ctrl Pts',(1.00891253001624,-0.609623316038242,
59.0151397869164));
#43210=CARTESIAN_POINT('Ctrl Pts',(1.1775654020451,-0.0537103769081715,
59.0389151522136));
#43211=CARTESIAN_POINT('Ctrl Pts',(1.060219428153,0.51524736277654,59.0626905175107));
#43212=CARTESIAN_POINT('Ctrl Pts',(0.685374777458641,0.959065427958262,
59.0864658828078));
#43213=CARTESIAN_POINT('Ctrl Pts',(0.144071096092974,1.16995239217321,59.110241248105));
#43214=CARTESIAN_POINT('Ctrl Pts',(-0.432223565087148,1.09668950503987,
59.1340166134021));
#43215=CARTESIAN_POINT('Ctrl Pts',(-0.903542790864627,0.757070343995723,
59.1577919786993));
#43216=CARTESIAN_POINT('Ctrl Pts',(-1.15541586530421,0.233579234703329,
59.1815673439965));
#43217=CARTESIAN_POINT('Ctrl Pts',(-1.12666961833547,-0.346641964858551,
59.2053427092936));
#43218=CARTESIAN_POINT('Ctrl Pts',(-0.82428573729697,-0.842673189303012,
59.2291180745908));
#43219=CARTESIAN_POINT('Ctrl Pts',(-0.321705103562753,-1.13404184535795,
59.2528934398879));
#43220=CARTESIAN_POINT('Ctrl Pts',(0.259009014889653,-1.14998235242418,
59.2766688051851));
#43221=CARTESIAN_POINT('Ctrl Pts',(0.776816835983212,-0.886623191674403,
59.3004441704823));
#43222=CARTESIAN_POINT('Ctrl Pts',(1.10595681901059,-0.407927193458844,
59.3242195357794));
#43223=CARTESIAN_POINT('Ctrl Pts',(1.16648974775348,0.16984330740993,59.3479949010765));
#43224=CARTESIAN_POINT('Ctrl Pts',(0.94371380798938,0.706363454096405,59.3717702663737));
#43225=CARTESIAN_POINT('Ctrl Pts',(0.491735261326532,1.0713269871797,59.3955456316708));
#43226=CARTESIAN_POINT('Ctrl Pts',(-0.0796725051838685,1.17609411723707,
59.419320996968));
#43227=CARTESIAN_POINT('Ctrl Pts',(-0.631729970982799,0.995219736738363,
59.4430963622652));
#43228=CARTESIAN_POINT('Ctrl Pts',(-1.03035728156532,0.572633349702764,
59.4668717275623));
#43229=CARTESIAN_POINT('Ctrl Pts',(-1.17873862417058,0.0109697811866665,
59.4906470928595));
#43230=CARTESIAN_POINT('Ctrl Pts',(-1.04083617774728,-0.553358051079711,
59.5144224581566));
#43231=CARTESIAN_POINT('Ctrl Pts',(-0.650142720880909,-0.983290151411998,
59.5381978234538));
#43232=CARTESIAN_POINT('Ctrl Pts',(-0.101547152799094,-1.17440761965159,
59.5619731887509));
#43233=CARTESIAN_POINT('Ctrl Pts',(0.471711486017707,-1.08029318159782,
59.5857485540481));
#43234=CARTESIAN_POINT('Ctrl Pts',(0.93040412062756,-0.723804694957189,
59.6095239193452));
#43235=CARTESIAN_POINT('Ctrl Pts',(1.16312675268372,-0.191523585992356,
59.6332992846424));
#43236=CARTESIAN_POINT('Ctrl Pts',(1.11335720939914,0.387273426872361,59.6570746499396));
#43237=CARTESIAN_POINT('Ctrl Pts',(0.793183445420126,0.872012189522576,
59.6808500152367));
#43238=CARTESIAN_POINT('Ctrl Pts',(0.280366428967129,1.14496271124877,59.7046253805339));
#43239=CARTESIAN_POINT('Ctrl Pts',(-0.300543148672945,1.13983274835279,
59.728400745831));
#43240=CARTESIAN_POINT('Ctrl Pts',(-0.808460801791496,0.857868086924541,
59.7521761111282));
#43241=CARTESIAN_POINT('Ctrl Pts',(-1.12002109956608,0.367550667285518,
59.7759514764253));
#43242=CARTESIAN_POINT('Ctrl Pts',(-1.15956736401967,-0.212035247289841,
59.7997268417224));
#43243=CARTESIAN_POINT('Ctrl Pts',(-0.917467489156749,-0.740122028302085,
59.8235022070197));
#43244=CARTESIAN_POINT('Ctrl Pts',(-0.452582019722852,-1.0884530823275,
59.8472775723168));
#43245=CARTESIAN_POINT('Ctrl Pts',(0.122304101199269,-1.17241375087369,
59.871052937614));
#43246=CARTESIAN_POINT('Ctrl Pts',(0.485598392798923,-1.03852712465534,
59.8869031811454));
#43247=CARTESIAN_POINT('Ctrl Pts',(0.64033508002711,-0.932242155189131,
59.8948283029111));
#43248=CARTESIAN_POINT('Ctrl Pts',(0.623398732068366,-0.874219306856439,
56.0287216970889));
#43249=CARTESIAN_POINT('Ctrl Pts',(0.768504591850525,-0.770745489366451,
56.0366468188546));
#43250=CARTESIAN_POINT('Ctrl Pts',(1.00602699863118,-0.490212309141386,
56.0524970623861));
#43251=CARTESIAN_POINT('Ctrl Pts',(1.11801361188198,0.0498751246670368,
56.0762724276832));
#43252=CARTESIAN_POINT('Ctrl Pts',(0.958425720631955,0.577781974785802,
56.1000477929803));
#43253=CARTESIAN_POINT('Ctrl Pts',(0.566075848520809,0.965399103995967,
56.1238231582775));
#43254=CARTESIAN_POINT('Ctrl Pts',(0.0362340764180832,1.11853081022668,
56.1475985235747));
#43255=CARTESIAN_POINT('Ctrl Pts',(-0.502404774606105,1.00000936060083,
56.1713738888718));
#43256=CARTESIAN_POINT('Ctrl Pts',(-0.919024600976301,0.638609097738095,
56.195149254169));
#43257=CARTESIAN_POINT('Ctrl Pts',(-1.11243746181925,0.122109582471567,
56.2189246194661));
#43258=CARTESIAN_POINT('Ctrl Pts',(-1.03566962247792,-0.424047819194122,
56.2426999847633));
#43259=CARTESIAN_POINT('Ctrl Pts',(-0.707365440007877,-0.867215097504543,
56.2664753500605));
#43260=CARTESIAN_POINT('Ctrl Pts',(-0.207261358948599,-1.0997594054429,
56.2902507153576));
#43261=CARTESIAN_POINT('Ctrl Pts',(0.343180943467093,-1.06520176695407,
56.3140260806547));
#43262=CARTESIAN_POINT('Ctrl Pts',(0.81027384428683,-0.771935411601755,
56.3378014459519));
#43263=CARTESIAN_POINT('Ctrl Pts',(1.08057310997332,-0.291186767898998,
56.3615768112491));
#43264=CARTESIAN_POINT('Ctrl Pts',(1.08843033576408,0.260283273030794,56.3853521765462));
#43265=CARTESIAN_POINT('Ctrl Pts',(0.83193721840397,0.748537537248444,56.4091275418434));
#43266=CARTESIAN_POINT('Ctrl Pts',(0.373389009449589,1.05499223997325,56.4329029071405));
#43267=CARTESIAN_POINT('Ctrl Pts',(-0.175845309349143,1.10521780955267,
56.4566782724377));
#43268=CARTESIAN_POINT('Ctrl Pts',(-0.682371549879583,0.887015809935557,
56.4804536377348));
#43269=CARTESIAN_POINT('Ctrl Pts',(-1.0231681625707,0.45338161664081,56.504229003032));
#43270=CARTESIAN_POINT('Ctrl Pts',(-1.11546485064466,-0.0903667316603153,
56.5280043683291));
#43271=CARTESIAN_POINT('Ctrl Pts',(-0.936845240215391,-0.612167440398215,
56.5517797336263));
#43272=CARTESIAN_POINT('Ctrl Pts',(-0.530691212560068,-0.985289204305658,
56.5755550989234));
#43273=CARTESIAN_POINT('Ctrl Pts',(0.00435338378282068,-1.11911081991613,
56.5993304642206));
#43274=CARTESIAN_POINT('Ctrl Pts',(0.538340660729817,-0.98113062953466,
56.6231058295177));
#43275=CARTESIAN_POINT('Ctrl Pts',(0.941579524541688,-0.60486029640679,
56.6468811948149));
#43276=CARTESIAN_POINT('Ctrl Pts',(1.1161341412668,-0.0816857264404262,
56.6706565601121));
#43277=CARTESIAN_POINT('Ctrl Pts',(1.01960990688035,0.461328101243613,56.6944319254092));
#43278=CARTESIAN_POINT('Ctrl Pts',(0.675449952090617,0.892297787415319,
56.7182072907064));
#43279=CARTESIAN_POINT('Ctrl Pts',(0.167241438775177,1.10655243001042,56.7419826560035));
#43280=CARTESIAN_POINT('Ctrl Pts',(-0.381585505072281,1.05205536048454,
56.7657580213007));
#43281=CARTESIAN_POINT('Ctrl Pts',(-0.837735631240389,0.742042445791208,
56.7895333865978));
#43282=CARTESIAN_POINT('Ctrl Pts',(-1.09042238857522,0.251807453621685,
56.813308751895));
#43283=CARTESIAN_POINT('Ctrl Pts',(-1.07827498539781,-0.299584771093069,
56.8370841171922));
#43284=CARTESIAN_POINT('Ctrl Pts',(-0.804243698001629,-0.778215942672852,
56.8608594824893));
#43285=CARTESIAN_POINT('Ctrl Pts',(-0.334883328188288,-1.06783947094452,
56.8846348477864));
#43286=CARTESIAN_POINT('Ctrl Pts',(0.215811161338217,-1.09811361973494,
56.9084102130836));
#43287=CARTESIAN_POINT('Ctrl Pts',(0.714090945938441,-0.861685615601347,
56.9321855783807));
#43288=CARTESIAN_POINT('Ctrl Pts',(1.03893731778188,-0.415977438000807,
56.9559609436779));
#43289=CARTESIAN_POINT('Ctrl Pts',(1.11145386288807,0.130760429322928,56.979736308975));
#43290=CARTESIAN_POINT('Ctrl Pts',(0.914028270149248,0.645740118448208,
57.0035116742722));
#43291=CARTESIAN_POINT('Ctrl Pts',(0.494609886226332,1.00388696557566,57.0272870395693));
#43292=CARTESIAN_POINT('Ctrl Pts',(-0.0449358862867625,1.11821677027719,
57.0510624048665));
#43293=CARTESIAN_POINT('Ctrl Pts',(-0.573567945135943,0.960961909504253,
57.0748377701637));
#43294=CARTESIAN_POINT('Ctrl Pts',(-0.962895834483168,0.570315343595536,
57.0986131354608));
#43295=CARTESIAN_POINT('Ctrl Pts',(-1.11836232052659,0.0411545772899142,
57.122388500758));
#43296=CARTESIAN_POINT('Ctrl Pts',(-1.00220879086932,-0.498001524806689,
57.1461638660551));
#43297=CARTESIAN_POINT('Ctrl Pts',(-0.642645802117325,-0.916206500864576,
57.1699392313523));
#43298=CARTESIAN_POINT('Ctrl Pts',(-0.127001497268327,-1.11188965230239,
57.1937145966494));
#43299=CARTESIAN_POINT('Ctrl Pts',(0.419488042661364,-1.03752482441128,
57.2174899619466));
#43300=CARTESIAN_POINT('Ctrl Pts',(0.864095261770125,-0.711173226290157,
57.2412653272438));
#43301=CARTESIAN_POINT('Ctrl Pts',(1.09883706940975,-0.212096850746369,
57.2650406925409));
#43302=CARTESIAN_POINT('Ctrl Pts',(1.06670101773,0.338492123954616,57.2888160578381));
#43303=CARTESIAN_POINT('Ctrl Pts',(0.775492086120482,0.80687049987593,57.3125914231352));
#43304=CARTESIAN_POINT('Ctrl Pts',(0.295937062424609,1.07928181411947,57.3363667884324));
#43305=CARTESIAN_POINT('Ctrl Pts',(-0.255493084446318,1.08956471262869,
57.3601421537295));
#43306=CARTESIAN_POINT('Ctrl Pts',(-0.744870858544122,0.835221756958756,
57.3839175190267));
#43307=CARTESIAN_POINT('Ctrl Pts',(-1.05333961006553,0.378025984652554,
57.4076928843238));
#43308=CARTESIAN_POINT('Ctrl Pts',(-1.10598060686658,-0.17098209391791,
57.431468249621));
#43309=CARTESIAN_POINT('Ctrl Pts',(-0.890008771951069,-0.678463237807091,
57.4552436149181));
#43310=CARTESIAN_POINT('Ctrl Pts',(-0.457877833519551,-1.0211639774184,
57.4790189802153));
#43311=CARTESIAN_POINT('Ctrl Pts',(0.0854592695393839,-1.11585155484739,
57.5027943455124));
#43312=CARTESIAN_POINT('Ctrl Pts',(0.608040623135005,-0.939528913777072,
57.5265697108096));
#43313=CARTESIAN_POINT('Ctrl Pts',(0.982945324387024,-0.535020063615578,
57.5503450761068));
#43314=CARTESIAN_POINT('Ctrl Pts',(1.1191191425052,-0.000569283712549584,
57.5741204414039));
#43315=CARTESIAN_POINT('Ctrl Pts',(0.983489133295694,0.534019759835548,
57.5978958067011));
#43316=CARTESIAN_POINT('Ctrl Pts',(0.608996164449402,0.938909820425502,
57.6216711719982));
#43317=CARTESIAN_POINT('Ctrl Pts',(0.0865944680705869,1.11576403298596,
57.6454465372954));
#43318=CARTESIAN_POINT('Ctrl Pts',(-0.456838686848294,1.02162928374448,
57.6692219025925));
#43319=CARTESIAN_POINT('Ctrl Pts',(-0.889318057812799,0.67936836197574,
57.6929972678897));
#43320=CARTESIAN_POINT('Ctrl Pts',(-1.10580608107857,0.172107205703827,
57.7167726331868));
#43321=CARTESIAN_POINT('Ctrl Pts',(-1.05372366023009,-0.376954144528003,
57.740547998484));
#43322=CARTESIAN_POINT('Ctrl Pts',(-0.74572020924432,-0.834463509525814,
57.7643233637811));
#43323=CARTESIAN_POINT('Ctrl Pts',(-0.256601451326632,-1.08930421571873,
57.7880987290783));
#43324=CARTESIAN_POINT('Ctrl Pts',(0.294838871757291,-1.0795823353994,57.8118740943754));
#43325=CARTESIAN_POINT('Ctrl Pts',(0.774670792531859,-0.80765905083989,
57.8356494596726));
#43326=CARTESIAN_POINT('Ctrl Pts',(1.06635609126063,-0.339577186861649,
57.8594248249698));
#43327=CARTESIAN_POINT('Ctrl Pts',(1.09905228338722,0.210978808383394,57.8832001902669));
#43328=CARTESIAN_POINT('Ctrl Pts',(0.864818346529344,0.710293746777896,
57.9069755555641));
#43329=CARTESIAN_POINT('Ctrl Pts',(0.420543380435131,1.03709750958033,57.9307509208612));
#43330=CARTESIAN_POINT('Ctrl Pts',(-0.125870219534756,1.11201828538914,
57.9545262861584));
#43331=CARTESIAN_POINT('Ctrl Pts',(-0.641713341244805,0.916859840364906,
57.9783016514555));
#43332=CARTESIAN_POINT('Ctrl Pts',(-1.00170161643053,0.4990208921939,58.0020770167527));
#43333=CARTESIAN_POINT('Ctrl Pts',(-1.11840361150074,-0.0400167588347418,
58.0258523820498));
#43334=CARTESIAN_POINT('Ctrl Pts',(-0.96347556240735,-0.569335419457958,
58.049627747347));
#43335=CARTESIAN_POINT('Ctrl Pts',(-0.574545309748047,-0.960377876802694,
58.0734031126442));
#43336=CARTESIAN_POINT('Ctrl Pts',(-0.0460735121080044,-1.11817047478798,
58.0971784779413));
#43337=CARTESIAN_POINT('Ctrl Pts',(0.493588297795928,-1.00438965122329,
58.1209538432384));
#43338=CARTESIAN_POINT('Ctrl Pts',(0.913370835360033,-0.646669696459674,
58.1447292085356));
#43339=CARTESIAN_POINT('Ctrl Pts',(1.11132025490185,-0.13189113029467,58.1685045738328));
#43340=CARTESIAN_POINT('Ctrl Pts',(1.03935998637156,0.414920230809768,58.1922799391299));
#43341=CARTESIAN_POINT('Ctrl Pts',(0.714967236314193,0.86095866927674,58.2160553044271));
#43342=CARTESIAN_POINT('Ctrl Pts',(0.216928246224609,1.09789348991396,58.2398306697243));
#43343=CARTESIAN_POINT('Ctrl Pts',(-0.333796758552693,1.06817962121791,
58.2636060350214));
#43344=CARTESIAN_POINT('Ctrl Pts',(-0.803451542047654,0.779033759722117,
58.2873814003185));
#43345=CARTESIAN_POINT('Ctrl Pts',(-1.07796963642117,0.300681629235197,
58.3111567656157));
#43346=CARTESIAN_POINT('Ctrl Pts',(-1.09067800759897,-0.250697951618005,
58.3349321309128));
#43347=CARTESIAN_POINT('Ctrl Pts',(-0.838490135304495,-0.741189768009906,
58.35870749621));
#43348=CARTESIAN_POINT('Ctrl Pts',(-0.382655645508598,-1.05166659933932,
58.3824828615072));
#43349=CARTESIAN_POINT('Ctrl Pts',(0.166115570188494,-1.10672200508822,
58.4062582268043));
#43350=CARTESIAN_POINT('Ctrl Pts',(0.674541798438691,-0.892984513507725,
58.4300335921015));
#43351=CARTESIAN_POINT('Ctrl Pts',(1.01914003416817,-0.462365191121956,
58.4538089573986));
#43352=CARTESIAN_POINT('Ctrl Pts',(1.11621666889125,0.0805501539095563,
58.4775843226958));
#43353=CARTESIAN_POINT('Ctrl Pts',(0.942194408770615,0.603902041134919,
58.5013596879929));
#43354=CARTESIAN_POINT('Ctrl Pts',(0.53933856278411,0.980582425856949,58.5251350532901));
#43355=CARTESIAN_POINT('Ctrl Pts',(0.00549194019273262,1.11910581170792,
58.5489104185872));
#43356=CARTESIAN_POINT('Ctrl Pts',(-0.529688526407874,0.985828607921979,
58.5726857838844));
#43357=CARTESIAN_POINT('Ctrl Pts',(-0.936221949721437,0.613120249270339,
58.5964611491816));
#43358=CARTESIAN_POINT('Ctrl Pts',(-1.11537233623622,0.0915015342193444,
58.6202365144787));
#43359=CARTESIAN_POINT('Ctrl Pts',(-1.02362889351509,-0.452340433265256,
58.6440118797759));
#43360=CARTESIAN_POINT('Ctrl Pts',(-0.683273627036049,-0.886321121153351,
58.667787245073));
#43361=CARTESIAN_POINT('Ctrl Pts',(-0.176969642599475,-1.10503833635026,
58.6915626103702));
#43362=CARTESIAN_POINT('Ctrl Pts',(0.372315490449813,-1.05537157190093,
58.7153379756673));
#43363=CARTESIAN_POINT('Ctrl Pts',(0.831175242112888,-0.749383544057456,
58.7391133409645));
#43364=CARTESIAN_POINT('Ctrl Pts',(1.0881649663537,-0.261390484153449,58.7628887062616));
#43365=CARTESIAN_POINT('Ctrl Pts',(1.0808687969972,0.290087267702929,58.7866640715588));
#43366=CARTESIAN_POINT('Ctrl Pts',(0.811058776608478,0.771110653597713,
58.8104394368559));
#43367=CARTESIAN_POINT('Ctrl Pts',(0.344264475192786,1.06485207908224,58.8342148021531));
#43368=CARTESIAN_POINT('Ctrl Pts',(-0.206142373284595,1.09996968191952,
58.8579901674502));
#43369=CARTESIAN_POINT('Ctrl Pts',(-0.706482804429733,0.867934344435469,
58.8817655327474));
#43370=CARTESIAN_POINT('Ctrl Pts',(-1.03523763499677,0.425101185944966,
58.9055408980446));
#43371=CARTESIAN_POINT('Ctrl Pts',(-1.11256119189629,-0.120977574334403,
58.9293162633417));
#43372=CARTESIAN_POINT('Ctrl Pts',(-0.919673670628794,-0.637674147788424,
58.9530916286389));
#43373=CARTESIAN_POINT('Ctrl Pts',(-0.503422242807215,-0.999496885764276,
58.976866993936));
#43374=CARTESIAN_POINT('Ctrl Pts',(0.0350968571145739,-1.11856881318326,
59.0006423592332));
#43375=CARTESIAN_POINT('Ctrl Pts',(0.565091877938255,-0.965970573409845,
59.0244177245303));
#43376=CARTESIAN_POINT('Ctrl Pts',(0.957841337157492,-0.578764159254765,
59.0481930898275));
#43377=CARTESIAN_POINT('Ctrl Pts',(1.11795699401921,-0.050991555468266,
59.0719684551247));
#43378=CARTESIAN_POINT('Ctrl Pts',(1.00655107804644,0.489165520543995,59.0957438204218));
#43379=CARTESIAN_POINT('Ctrl Pts',(0.650681078650523,0.910517497411072,
59.119519185719));
#43380=CARTESIAN_POINT('Ctrl Pts',(0.136778211412653,1.11072935501331,59.1432945510161));
#43381=CARTESIAN_POINT('Ctrl Pts',(-0.410344390833752,1.04117503817409,
59.1670699163132));
#43382=CARTESIAN_POINT('Ctrl Pts',(-0.857805418440835,0.71874741272513,
59.1908452816104));
#43383=CARTESIAN_POINT('Ctrl Pts',(-1.09692866771924,0.221755444445569,
59.2146206469076));
#43384=CARTESIAN_POINT('Ctrl Pts',(-1.06963755692854,-0.32909493465174,
59.2383960122047));
#43385=CARTESIAN_POINT('Ctrl Pts',(-0.782560360113341,-0.800017038559101,
59.2621713775019));
#43386=CARTESIAN_POINT('Ctrl Pts',(-0.305420378277957,-1.07663660152255,
59.2859467427991));
#43387=CARTESIAN_POINT('Ctrl Pts',(0.245897968135809,-1.09177019947979,
59.3097221080962));
#43388=CARTESIAN_POINT('Ctrl Pts',(0.737494336493802,-0.841742290042304,
59.3334974733934));
#43389=CARTESIAN_POINT('Ctrl Pts',(1.04997324033878,-0.387277902514728,
59.3572728386905));
#43390=CARTESIAN_POINT('Ctrl Pts',(1.10744198979342,0.161245832355916,59.3810482039877));
#43391=CARTESIAN_POINT('Ctrl Pts',(0.895942977062618,0.670607307632499,
59.4048235692848));
#43392=CARTESIAN_POINT('Ctrl Pts',(0.466843602615289,1.01709637198835,59.428598934582));
#43393=CARTESIAN_POINT('Ctrl Pts',(-0.0756394797661783,1.11656018570735,
59.4523742998791));
#43394=CARTESIAN_POINT('Ctrl Pts',(-0.599751774436666,0.944841673626204,
59.4761496651763));
#43395=CARTESIAN_POINT('Ctrl Pts',(-0.978200554520414,0.543646626503323,
59.4999250304734));
#43396=CARTESIAN_POINT('Ctrl Pts',(-1.1190708275935,0.0104144904216708,
59.5237003957706));
#43397=CARTESIAN_POINT('Ctrl Pts',(-0.988149008556066,-0.525347044272036,
59.5474757610677));
#43398=CARTESIAN_POINT('Ctrl Pts',(-0.617232470194169,-0.933515964389,59.5712511263649));
#43399=CARTESIAN_POINT('Ctrl Pts',(-0.0964068318390796,-1.1149590586975,
59.595026491662));
#43400=CARTESIAN_POINT('Ctrl Pts',(0.447833431618176,-1.02560869728431,
59.6188018569592));
#43401=CARTESIAN_POINT('Ctrl Pts',(0.883307026610518,-0.68716567217923,
59.6425772222563));
#43402=CARTESIAN_POINT('Ctrl Pts',(1.10424922966938,-0.181828654364277,
59.6663525875535));
#43403=CARTESIAN_POINT('Ctrl Pts',(1.05699902266814,0.367669630423775,59.6901279528507));
#43404=CARTESIAN_POINT('Ctrl Pts',(0.753032467502573,0.827870897407221,
59.7139033181478));
#43405=CARTESIAN_POINT('Ctrl Pts',(0.266174269053451,1.08700465274262,59.737678683445));
#43406=CARTESIAN_POINT('Ctrl Pts',(-0.285329642396041,1.08213436877481,
59.7614540487421));
#43407=CARTESIAN_POINT('Ctrl Pts',(-0.76753648347981,0.814442769851721,
59.7852294140393));
#43408=CARTESIAN_POINT('Ctrl Pts',(-1.06332558644673,0.348945237720674,
59.8090047793364));
#43409=CARTESIAN_POINT('Ctrl Pts',(-1.1008700174027,-0.201302014541691,
59.8327801446336));
#43410=CARTESIAN_POINT('Ctrl Pts',(-0.871025247945204,-0.702657021453754,
59.8565555099308));
#43411=CARTESIAN_POINT('Ctrl Pts',(-0.429672299676753,-1.03335554351077,
59.8803308752279));
#43412=CARTESIAN_POINT('Ctrl Pts',(0.116113062676177,-1.11306611963735,
59.904106240525));
#43413=CARTESIAN_POINT('Ctrl Pts',(0.461017382619445,-0.985956839824536,
59.9199564840565));
#43414=CARTESIAN_POINT('Ctrl Pts',(0.607921292514964,-0.885052019788631,
59.9278816058222));
#43415=CARTESIAN_POINT('Ctrl Pts',(0.590159702138998,-0.827606761449064,
56.061775));
#43416=CARTESIAN_POINT('Ctrl Pts',(0.727528654917474,-0.729650069900356,
56.0697001217657));
#43417=CARTESIAN_POINT('Ctrl Pts',(0.952386591942655,-0.464074653132307,
56.0855503652972));
#43418=CARTESIAN_POINT('Ctrl Pts',(1.05840218504528,0.0472158302600112,
56.1093257305943));
#43419=CARTESIAN_POINT('Ctrl Pts',(0.907323368999851,0.546975187147921,
56.1331010958915));
#43420=CARTESIAN_POINT('Ctrl Pts',(0.535893220447681,0.913924938167876,
56.1568764611886));
#43421=CARTESIAN_POINT('Ctrl Pts',(0.0343021097832936,1.05889180686411,
56.1806518264858));
#43422=CARTESIAN_POINT('Ctrl Pts',(-0.475617027886791,0.946689808672358,
56.2044271917829));
#43423=CARTESIAN_POINT('Ctrl Pts',(-0.870023079724685,0.604559065518011,
56.22820255708));
#43424=CARTESIAN_POINT('Ctrl Pts',(-1.05312335002233,0.1155988151927,56.2519779223772));
#43425=CARTESIAN_POINT('Ctrl Pts',(-0.980448699162488,-0.401437991120026,
56.2757532876744));
#43426=CARTESIAN_POINT('Ctrl Pts',(-0.669649384741906,-0.820976009905639,
56.2995286529715));
#43427=CARTESIAN_POINT('Ctrl Pts',(-0.196210379601176,-1.04112127560369,
56.3233040182687));
#43428=CARTESIAN_POINT('Ctrl Pts',(0.324882860612091,-1.00840621766713,
56.3470793835659));
#43429=CARTESIAN_POINT('Ctrl Pts',(0.767070810376454,-0.730776546609132,
56.370854748863));
#43430=CARTESIAN_POINT('Ctrl Pts',(1.02295797523586,-0.275660965237961,
56.3946301141602));
#43431=CARTESIAN_POINT('Ctrl Pts',(1.03039626118959,0.246405215445278,56.4184054794573));
#43432=CARTESIAN_POINT('Ctrl Pts',(0.787579113904559,0.708626224754583,
56.4421808447545));
#43433=CARTESIAN_POINT('Ctrl Pts',(0.353480261128564,0.998741052994776,
56.4659562100516));
#43434=CARTESIAN_POINT('Ctrl Pts',(-0.166469404010035,1.04628864277636,
56.4897315753488));
#43435=CARTESIAN_POINT('Ctrl Pts',(-0.645988145161798,0.839720967104466,
56.5135069406459));
#43436=CARTESIAN_POINT('Ctrl Pts',(-0.968613805256519,0.429207738270938,
56.5372823059431));
#43437=CARTESIAN_POINT('Ctrl Pts',(-1.05598932134302,-0.0855484631208394,
56.5610576712402));
#43438=CARTESIAN_POINT('Ctrl Pts',(-0.886893539358715,-0.579527252302758,
56.5848330365374));
#43439=CARTESIAN_POINT('Ctrl Pts',(-0.502395259761104,-0.932754517168359,
56.6086084018346));
#43440=CARTESIAN_POINT('Ctrl Pts',(0.00412126548291853,-1.05944089098629,
56.6323837671317));
#43441=CARTESIAN_POINT('Ctrl Pts',(0.509636846599777,-0.928817673665269,
56.6561591324289));
#43442=CARTESIAN_POINT('Ctrl Pts',(0.89137539612891,-0.572609718307843,
56.679934497726));
#43443=CARTESIAN_POINT('Ctrl Pts',(1.05662292602311,-0.0773303208768799,
56.7037098630232));
#43444=CARTESIAN_POINT('Ctrl Pts',(0.965245272389302,0.436730523841399,
56.7274852283203));
#43445=CARTESIAN_POINT('Ctrl Pts',(0.639435600411005,0.844721314547941,
56.7512605936175));
#43446=CARTESIAN_POINT('Ctrl Pts',(0.158324283665738,1.04755210253542,56.7750359589146));
#43447=CARTESIAN_POINT('Ctrl Pts',(-0.361239727368135,0.995960765138673,
56.7988113242118));
#43448=CARTESIAN_POINT('Ctrl Pts',(-0.793068360860628,0.702477445421887,
56.8225866895089));
#43449=CARTESIAN_POINT('Ctrl Pts',(-1.03228209963166,0.238381318699013,
56.8463620548061));
#43450=CARTESIAN_POINT('Ctrl Pts',(-1.02078238448601,-0.283611194856068,
56.8701374201032));
#43451=CARTESIAN_POINT('Ctrl Pts',(-0.761362185779602,-0.736722205712254,
56.8939127854004));
#43452=CARTESIAN_POINT('Ctrl Pts',(-0.317027666320693,-1.01090328177916,
56.9176881506975));
#43453=CARTESIAN_POINT('Ctrl Pts',(0.204304314625503,-1.03956324163084,
56.9414635159947));
#43454=CARTESIAN_POINT('Ctrl Pts',(0.676016293066456,-0.815741354740158,
56.9652388812919));
#43455=CARTESIAN_POINT('Ctrl Pts',(0.98354216404791,-0.393797915007909,
56.989014246589));
#43456=CARTESIAN_POINT('Ctrl Pts',(1.05219219565452,0.123788407083776,57.0127896118862));
#43457=CARTESIAN_POINT('Ctrl Pts',(0.865293148524952,0.611309866958155,
57.0365649771833));
#43458=CARTESIAN_POINT('Ctrl Pts',(0.468237755572337,0.950360663422683,
57.0603403424805));
#43459=CARTESIAN_POINT('Ctrl Pts',(-0.0425399473918753,1.05859451122728,
57.0841157077776));
#43460=CARTESIAN_POINT('Ctrl Pts',(-0.54298584556759,0.90972433068368,57.1078910730748));
#43461=CARTESIAN_POINT('Ctrl Pts',(-0.911555140614478,0.539906669660545,
57.1316664383719));
#43462=CARTESIAN_POINT('Ctrl Pts',(-1.05873230087524,0.0389602542091891,
57.1554418036691));
#43463=CARTESIAN_POINT('Ctrl Pts',(-0.948771967402165,-0.471448555196054,
57.1792171689663));
#43464=CARTESIAN_POINT('Ctrl Pts',(-0.608380536643186,-0.867355238041698,
57.2029925342634));
#43465=CARTESIAN_POINT('Ctrl Pts',(-0.120229897725971,-1.05260474919004,
57.2267678995606));
#43466=CARTESIAN_POINT('Ctrl Pts',(0.397121337553111,-0.982204983485956,
57.2505432648577));
#43467=CARTESIAN_POINT('Ctrl Pts',(0.818022520857566,-0.673254143466235,
57.2743186301549));
#43468=CARTESIAN_POINT('Ctrl Pts',(1.04024811765422,-0.200788047556321,
57.298093995452));
#43469=CARTESIAN_POINT('Ctrl Pts',(1.00982552981173,0.320444044514911,57.3218693607492));
#43470=CARTESIAN_POINT('Ctrl Pts',(0.734143582611297,0.763848929065998,
57.3456447260463));
#43471=CARTESIAN_POINT('Ctrl Pts',(0.280157978558803,1.02173553005387,57.3694200913435));
#43472=CARTESIAN_POINT('Ctrl Pts',(-0.241870435179003,1.03147015415423,
57.3931954566406));
#43473=CARTESIAN_POINT('Ctrl Pts',(-0.705155049885808,0.79068852397462,
57.4169708219378));
#43474=CARTESIAN_POINT('Ctrl Pts',(-0.997176539748407,0.35786999720571,
57.440746187235));
#43475=CARTESIAN_POINT('Ctrl Pts',(-1.04701076846,-0.161865490619304,57.4645215525321));
#43476=CARTESIAN_POINT('Ctrl Pts',(-0.842554347220154,-0.642288220587176,
57.4882969178293));
#43477=CARTESIAN_POINT('Ctrl Pts',(-0.433464221124387,-0.966716481358237,
57.5120722831264));
#43478=CARTESIAN_POINT('Ctrl Pts',(0.0809026622319955,-1.05635540684393,
57.5358476484236));
#43479=CARTESIAN_POINT('Ctrl Pts',(0.575620473027226,-0.889434121987983,
57.5596230137207));
#43480=CARTESIAN_POINT('Ctrl Pts',(0.930535610706933,-0.506493300578492,
57.5833983790179));
#43481=CARTESIAN_POINT('Ctrl Pts',(1.05944876982279,-0.000538930044200919,
57.607173744315));
#43482=CARTESIAN_POINT('Ctrl Pts',(0.931050424239669,0.505546332048563,
57.6309491096122));
#43483=CARTESIAN_POINT('Ctrl Pts',(0.576525065783793,0.888848038107536,
57.6547244749094));
#43484=CARTESIAN_POINT('Ctrl Pts',(0.0819773330527327,1.05627255156526,
57.6784998402065));
#43485=CARTESIAN_POINT('Ctrl Pts',(-0.432480480769399,0.967156977991728,
57.7022752055036));
#43486=CARTESIAN_POINT('Ctrl Pts',(-0.841900461305519,0.643145084392453,
57.7260505708008));
#43487=CARTESIAN_POINT('Ctrl Pts',(-1.0468455482217,0.16293061251046,57.7498259360979));
#43488=CARTESIAN_POINT('Ctrl Pts',(-0.99754011272195,-0.356855306581392,
57.7736013013951));
#43489=CARTESIAN_POINT('Ctrl Pts',(-0.705959114011145,-0.789970705576619,
57.7973766666922));
#43490=CARTESIAN_POINT('Ctrl Pts',(-0.242919704987064,-1.03122354669277,
57.8211520319894));
#43491=CARTESIAN_POINT('Ctrl Pts',(0.2791183423777,-1.02202002782379,57.8449273972865));
#43492=CARTESIAN_POINT('Ctrl Pts',(0.73336607961892,-0.764595435239446,
57.8687027625837));
#43493=CARTESIAN_POINT('Ctrl Pts',(1.00949899449501,-0.321471252895473,
57.8924781278809));
#43494=CARTESIAN_POINT('Ctrl Pts',(1.04045185662625,0.199729618153172,57.916253493178));
#43495=CARTESIAN_POINT('Ctrl Pts',(0.818707051422304,0.672421556968558,
57.9400288584752));
#43496=CARTESIAN_POINT('Ctrl Pts',(0.398120405716357,0.981800452677053,
57.9638042237723));
#43497=CARTESIAN_POINT('Ctrl Pts',(-0.11915893864965,1.05272652368244,57.9875795890695));
#43498=CARTESIAN_POINT('Ctrl Pts',(-0.607497793701196,0.867973742098689,
58.0113549543666));
#43499=CARTESIAN_POINT('Ctrl Pts',(-0.948291835024074,0.472413570879686,
58.0351303196638));
#43500=CARTESIAN_POINT('Ctrl Pts',(-1.05877139025375,-0.0378831031563466,
58.058905684961));
#43501=CARTESIAN_POINT('Ctrl Pts',(-0.912103957994839,-0.538978994149835,
58.0826810502581));
#43502=CARTESIAN_POINT('Ctrl Pts',(-0.543911098024301,-0.909171438052593,
58.1064564155553));
#43503=CARTESIAN_POINT('Ctrl Pts',(-0.0436169160818455,-1.0585506841697,
58.1302317808524));
#43504=CARTESIAN_POINT('Ctrl Pts',(0.467270637269431,-0.950836546347711,
58.1540071461496));
#43505=CARTESIAN_POINT('Ctrl Pts',(0.864670767536001,-0.612189880750512,
58.1777825114467));
#43506=CARTESIAN_POINT('Ctrl Pts',(1.05206571151958,-0.124858820150662,
58.2015578767439));
#43507=CARTESIAN_POINT('Ctrl Pts',(0.983942296348724,0.392797077102948,
58.2253332420411));
#43508=CARTESIAN_POINT('Ctrl Pts',(0.676845860469362,0.815053168505043,
58.2491086073382));
#43509=CARTESIAN_POINT('Ctrl Pts',(0.205361837603814,1.03935484892341,58.2728839726354));
#43510=CARTESIAN_POINT('Ctrl Pts',(-0.315999031548909,1.01122529556216,
58.2966593379325));
#43511=CARTESIAN_POINT('Ctrl Pts',(-0.760612266830792,0.737496417531059,
58.3204347032296));
#43512=CARTESIAN_POINT('Ctrl Pts',(-1.02049331642759,0.28464956956096,58.3442100685268));
#43513=CARTESIAN_POINT('Ctrl Pts',(-1.03252408929118,-0.237330974291291,
58.367985433824));
#43514=CARTESIAN_POINT('Ctrl Pts',(-0.793782635482674,-0.701670231612259,
58.3917607991211));
#43515=CARTESIAN_POINT('Ctrl Pts',(-0.362252808929985,-0.995592732369494,
58.4155361644183));
#43516=CARTESIAN_POINT('Ctrl Pts',(0.157258445325715,-1.04771263603068,
58.4393115297154));
#43517=CARTESIAN_POINT('Ctrl Pts',(0.63857586865163,-0.845371425055543,
58.4630868950126));
#43518=CARTESIAN_POINT('Ctrl Pts',(0.964800452845084,-0.437712317069721,
58.4868622603097));
#43519=CARTESIAN_POINT('Ctrl Pts',(1.0567010533528,0.0762552959977839,58.5106376256069));
#43520=CARTESIAN_POINT('Ctrl Pts',(0.891957495313147,0.571702556299444,
58.534412990904));
#43521=CARTESIAN_POINT('Ctrl Pts',(0.51058154146171,0.928298699688416,58.5581883562012));
#43522=CARTESIAN_POINT('Ctrl Pts',(0.00519911514345259,1.059436149811,58.5819637214983));
#43523=CARTESIAN_POINT('Ctrl Pts',(-0.501446035884838,0.93326516029476,
58.6057390867955));
#43524=CARTESIAN_POINT('Ctrl Pts',(-0.886303482123542,0.580429258308285,
58.6295144520927));
#43525=CARTESIAN_POINT('Ctrl Pts',(-1.05590173971521,0.0866227590822638,
58.6532898173898));
#43526=CARTESIAN_POINT('Ctrl Pts',(-0.969049970463342,-0.428222069806799,
58.677065182687));
#43527=CARTESIAN_POINT('Ctrl Pts',(-0.646842124418696,-0.839063318470144,
58.7008405479841));
#43528=CARTESIAN_POINT('Ctrl Pts',(-0.167533788876386,-1.04611873891511,
58.7246159132813));
#43529=CARTESIAN_POINT('Ctrl Pts',(0.352463981145058,-0.999100159303358,
58.7483912785784));
#43530=CARTESIAN_POINT('Ctrl Pts',(0.786857765467602,-0.709427123281846,
58.7721666438756));
#43531=CARTESIAN_POINT('Ctrl Pts',(1.03014504102483,-0.247453391119582,
58.7959420091728));
#43532=CARTESIAN_POINT('Ctrl Pts',(1.0232378965077,0.274620089350941,58.8197173744699));
#43533=CARTESIAN_POINT('Ctrl Pts',(0.767813890850171,0.729995763920686,
58.8434927397671));
#43534=CARTESIAN_POINT('Ctrl Pts',(0.325908619452451,1.00807517482141,58.8672681050642));
#43535=CARTESIAN_POINT('Ctrl Pts',(-0.195151057192915,1.04132034033774,
58.8910434703614));
#43536=CARTESIAN_POINT('Ctrl Pts',(-0.66881381045679,0.821656907271453,
58.9148188356585));
#43537=CARTESIAN_POINT('Ctrl Pts',(-0.980039744844674,0.402435193353424,
58.9385942009557));
#43538=CARTESIAN_POINT('Ctrl Pts',(-1.05324048292885,-0.114527164657214,
58.9623695662528));
#43539=CARTESIAN_POINT('Ctrl Pts',(-0.870637541598082,-0.603673966214107,
58.98614493155));
#43540=CARTESIAN_POINT('Ctrl Pts',(-0.476580245647126,-0.946204658508691,
59.0099202968471));
#43541=CARTESIAN_POINT('Ctrl Pts',(0.0332255259359154,-1.05892778353904,
59.0336956621443));
#43542=CARTESIAN_POINT('Ctrl Pts',(0.534961714244608,-0.914465937373881,
59.0574710274415));
#43543=CARTESIAN_POINT('Ctrl Pts',(0.906770144298739,-0.547905002471288,
59.0812463927386));
#43544=CARTESIAN_POINT('Ctrl Pts',(1.05834858599332,-0.0482727340283605,
59.1050217580358));
#43545=CARTESIAN_POINT('Ctrl Pts',(0.952882727939887,0.463083678311449,
59.1287971233329));
#43546=CARTESIAN_POINT('Ctrl Pts',(0.615987379842406,0.861969566863883,
59.15257248863));
#43547=CARTESIAN_POINT('Ctrl Pts',(0.129485326732331,1.05150631785341,59.1763478539272));
#43548=CARTESIAN_POINT('Ctrl Pts',(-0.388465216580355,0.985660571308298,
59.2001232192243));
#43549=CARTESIAN_POINT('Ctrl Pts',(-0.812068046017044,0.680424481454538,
59.2238985845215));
#43550=CARTESIAN_POINT('Ctrl Pts',(-1.03844147013426,0.209931654187809,
59.2476739498187));
#43551=CARTESIAN_POINT('Ctrl Pts',(-1.01260549552161,-0.311547904444929,
59.2714493151158));
#43552=CARTESIAN_POINT('Ctrl Pts',(-0.740834982929712,-0.75736088781519,
59.295224680413));
#43553=CARTESIAN_POINT('Ctrl Pts',(-0.289135652993162,-1.01923135768715,
59.3190000457102));
#43554=CARTESIAN_POINT('Ctrl Pts',(0.232786921381965,-1.0335580465354,59.3427754110073));
#43555=CARTESIAN_POINT('Ctrl Pts',(0.698171837004391,-0.796861388410206,
59.3665507763045));
#43556=CARTESIAN_POINT('Ctrl Pts',(0.993989661666965,-0.36662861157061,
59.3903261416016));
#43557=CARTESIAN_POINT('Ctrl Pts',(1.04839423183335,0.152648357301901,59.4141015068988));
#43558=CARTESIAN_POINT('Ctrl Pts',(0.848172146135856,0.634851161168593,
59.4378768721959));
#43559=CARTESIAN_POINT('Ctrl Pts',(0.441951943904046,0.962865756797002,
59.4616522374931));
#43560=CARTESIAN_POINT('Ctrl Pts',(-0.0716064543484882,1.05702625417764,
59.4854276027902));
#43561=CARTESIAN_POINT('Ctrl Pts',(-0.567773577890534,0.894463610514046,
59.5092029680874));
#43562=CARTESIAN_POINT('Ctrl Pts',(-0.926043827475508,0.514659903303883,
59.5329783333845));
#43563=CARTESIAN_POINT('Ctrl Pts',(-1.05940303101641,0.00985919965667513,
59.5567536986817));
#43564=CARTESIAN_POINT('Ctrl Pts',(-0.935461839364852,-0.497336037464362,
59.5805290639788));
#43565=CARTESIAN_POINT('Ctrl Pts',(-0.584322219507429,-0.883741777366003,
59.604304429276));
#43566=CARTESIAN_POINT('Ctrl Pts',(-0.0912665108790651,-1.05551049774341,
59.6280797945731));
#43567=CARTESIAN_POINT('Ctrl Pts',(0.423955377218644,-0.970924212970794,
59.6518551598703));
#43568=CARTESIAN_POINT('Ctrl Pts',(0.836209932593474,-0.65052664940127,
59.6756305251674));
#43569=CARTESIAN_POINT('Ctrl Pts',(1.04537170665504,-0.172133722736198,
59.6994058904646));
#43570=CARTESIAN_POINT('Ctrl Pts',(1.00064083593713,0.348065833975191,59.7231812557618));
#43571=CARTESIAN_POINT('Ctrl Pts',(0.712881489585019,0.783729605291864,
59.7469566210589));
#43572=CARTESIAN_POINT('Ctrl Pts',(0.251982109139772,1.02904659423647,59.7707319863561));
#43573=CARTESIAN_POINT('Ctrl Pts',(-0.270116136119136,1.02443598919684,
59.7945073516532));
#43574=CARTESIAN_POINT('Ctrl Pts',(-0.726612165168123,0.7710174527789,59.8182827169504));
#43575=CARTESIAN_POINT('Ctrl Pts',(-1.00663007332738,0.330339808155829,
59.8420580822475));
#43576=CARTESIAN_POINT('Ctrl Pts',(-1.04217267078573,-0.19056878179354,
59.8658334475447));
#43577=CARTESIAN_POINT('Ctrl Pts',(-0.82458300673366,-0.665192014605423,
59.8896088128418));
#43578=CARTESIAN_POINT('Ctrl Pts',(-0.406762579630654,-0.978258004694046,
59.913384178139));
#43579=CARTESIAN_POINT('Ctrl Pts',(0.109922024153085,-1.05371848840101,
59.9371595434362));
#43580=CARTESIAN_POINT('Ctrl Pts',(0.436436372439967,-0.933386554993731,
59.9530097869676));
#43581=CARTESIAN_POINT('Ctrl Pts',(0.575507505002819,-0.837861884388131,
59.9609349087333));
#43582=CARTESIAN_POINT('Ctrl Pts',(0.672748867539213,-0.979432290589659,
59.861775));
#43583=CARTESIAN_POINT('Ctrl Pts',(0.510179402978367,-1.09109740948616,
59.8538498782343));
#43584=CARTESIAN_POINT('Ctrl Pts',(0.319337271350366,-1.16142939579809,
59.8459247564686));
#43585=CARTESIAN_POINT('Ctrl Pts',(0.123251725621158,-1.18189359545975,
59.8379996347028));
#43586=CARTESIAN_POINT('Ctrl Pts',(-0.0728338201080729,-1.20235779512143,
59.8300745129371));
#43587=CARTESIAN_POINT('Ctrl Pts',(-0.274162779938513,-1.17295420813283,
59.8221493911714));
#43588=CARTESIAN_POINT('Ctrl Pts',(-0.456230258286956,-1.09725848363956,
59.8142242694057));
#43589=CARTESIAN_POINT('Ctrl Pts',(-0.638297736635399,-1.02156275914629,
59.80629914764));
#43590=CARTESIAN_POINT('Ctrl Pts',(-0.801103733501846,-0.899574897148353,
59.7983740258743));
#43591=CARTESIAN_POINT('Ctrl Pts',(-0.924899228646461,-0.74611120696398,
59.7904489041085));
#43592=CARTESIAN_POINT('Ctrl Pts',(-1.04869472379108,-0.592647516779607,
59.7825237823428));
#43593=CARTESIAN_POINT('Ctrl Pts',(-1.13347971721386,-0.407707998408799,
59.7745986605771));
#43594=CARTESIAN_POINT('Ctrl Pts',(-1.16894753093338,-0.213750809742003,
59.7666735388113));
#43595=CARTESIAN_POINT('Ctrl Pts',(-1.18182974287435,-0.143303907329611,
59.7637950671059));
#43596=CARTESIAN_POINT('Ctrl Pts',(-1.18820601150139,-0.0716673900178602,
59.7609165954006));
#43597=CARTESIAN_POINT('Ctrl Pts',(-1.18815715028295,-2.22996587661006E-5,
59.7580381236952));
#43598=CARTESIAN_POINT('Origin',(0.,0.,57.95));
#43599=CARTESIAN_POINT('Origin',(0.,0.,59.861775));
#43600=CARTESIAN_POINT('Origin',(1.7,0.,-23.));
#43601=CARTESIAN_POINT('',(-1.7,-2.0818995585505E-16,-23.));
#43602=CARTESIAN_POINT('Origin',(0.,0.,-23.));
#43603=CARTESIAN_POINT('Origin',(0.,0.,-22.85));
#43604=CARTESIAN_POINT('',(-2.,-2.4492935982947E-16,-22.7));
#43605=CARTESIAN_POINT('Origin',(0.,0.,-22.7));
#43606=CARTESIAN_POINT('',(-1.85,-2.2655965784226E-16,-22.85));
#43607=CARTESIAN_POINT('Origin',(0.,0.,16.65));
#43608=CARTESIAN_POINT('',(-2.,-2.44929359829471E-16,56.));
#43609=CARTESIAN_POINT('Origin',(0.,0.,56.));
#43610=CARTESIAN_POINT('',(-2.,-2.44929359829471E-16,16.65));
#43611=CARTESIAN_POINT('Origin',(1.25,0.,56.));
#43612=CARTESIAN_POINT('',(-1.25,-1.53080849893419E-16,56.));
#43613=CARTESIAN_POINT('Origin',(0.,0.,56.));
#43614=CARTESIAN_POINT('Origin',(0.,0.,56.025));
#43615=CARTESIAN_POINT('',(-1.225,-1.50019232895551E-16,56.025));
#43616=CARTESIAN_POINT('Origin',(0.,0.,59.925));
#43617=CARTESIAN_POINT('',(-1.05,-1.28587913910472E-16,60.));
#43618=CARTESIAN_POINT('Origin',(0.,0.,60.));
#43619=CARTESIAN_POINT('',(-1.125,-1.37772764904077E-16,59.925));
#43620=CARTESIAN_POINT('Origin',(0.,0.,60.));
#70726=UNCERTAINTY_MEASURE_WITH_UNIT(LENGTH_MEASURE(0.001),#70758,
'DISTANCE_ACCURACY_VALUE',
'Maximum model space distance between geometric entities at asserted c
onnectivities');
#70740=UNCERTAINTY_MEASURE_WITH_UNIT(LENGTH_MEASURE(0.001),#70758,
'DISTANCE_ACCURACY_VALUE',
'Maximum model space distance between geometric entities at asserted c
onnectivities');
#70743=(
GEOMETRIC_REPRESENTATION_CONTEXT(3)
GLOBAL_UNCERTAINTY_ASSIGNED_CONTEXT((#70726))
GLOBAL_UNIT_ASSIGNED_CONTEXT((#70758,#70760,#70761))
REPRESENTATION_CONTEXT('','3D')
);
#70757=(
GEOMETRIC_REPRESENTATION_CONTEXT(3)
GLOBAL_UNCERTAINTY_ASSIGNED_CONTEXT((#70740))
GLOBAL_UNIT_ASSIGNED_CONTEXT((#70758,#70760,#70761))
REPRESENTATION_CONTEXT('','3D')
);
#70758=(
LENGTH_UNIT()
NAMED_UNIT(*)
SI_UNIT(.CENTI.,.METRE.)
);
#70760=(
NAMED_UNIT(*)
PLANE_ANGLE_UNIT()
SI_UNIT($,.RADIAN.)
);
#70761=(
NAMED_UNIT(*)
SI_UNIT($,.STERADIAN.)
SOLID_ANGLE_UNIT()
);
#70764=SHAPE_DEFINITION_REPRESENTATION(#70780,#70819);
#70780=PRODUCT_DEFINITION_SHAPE('',$,#70836);
#70819=SHAPE_REPRESENTATION('',(#27231),#70743);
#70833=PRODUCT_DEFINITION_CONTEXT('part definition',#70883,'design');
#70836=PRODUCT_DEFINITION('2026-10-19-02-55-26-880',
'05_Operating_Lever_D40x790_M24_End',#70852,#70833);
#70852=PRODUCT_DEFINITION_FORMATION('',$,#70887);
#70883=APPLICATION_CONTEXT(
'Core Data for Automotive Mechanical Design Process');
#70884=PRODUCT_CONTEXT('part definition',#70883,'mechanical');
#70887=PRODUCT('2026-10-19-02-55-26-880',
'05_Operating_Lever_D40x790_M24_End',$,(#70884));
#71055=COLOUR_RGB('Off White',0.89,0.88,0.83);
#71056=FILL_AREA_STYLE_COLOUR('',#71055);
#71057=FILL_AREA_STYLE('',(#71056));
#71058=SURFACE_STYLE_FILL_AREA(#71057);
#71059=SURFACE_SIDE_STYLE('',(#71058));
#71060=SURFACE_STYLE_USAGE(.BOTH.,#71059);
#71061=PRESENTATION_STYLE_ASSIGNMENT((#71060));
ENDSEC;
END-ISO-10303-21;
